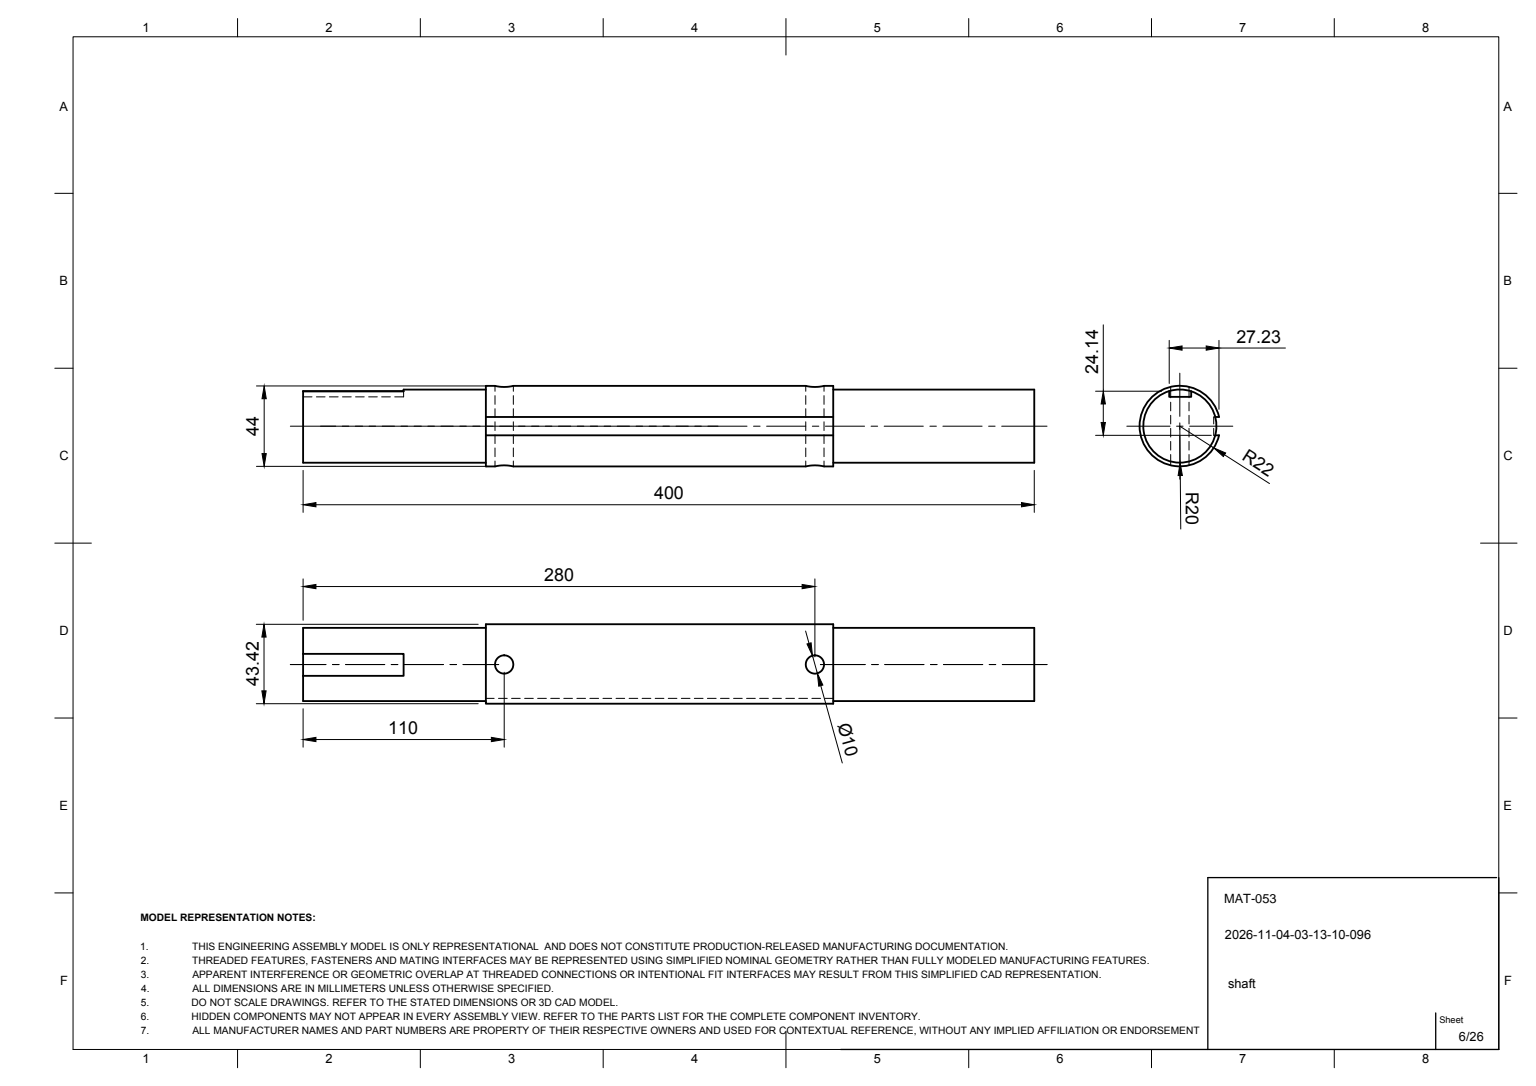
ISO-10303-21;
HEADER;
FILE_DESCRIPTION (('STEP AP214'),
    '1' );
FILE_NAME ('shaft.step',
    '2026-10-10T03:43:58',
    ( '' ),
    ( '' ),
    'SwSTEP 2.0',
    'SolidWorks 2026',
    '' );
FILE_SCHEMA (( 'AUTOMOTIVE_DESIGN' ));
ENDSEC;

DATA;
#13=ORIENTED_EDGE ( 'NONE', *, *, #19324, .T. ) ;
#42=CARTESIAN_POINT ( 'NONE',  ( 110.0000000000000284, 21.42428528562853174, 5.000000000000004441 ) ) ;
#241=DIRECTION ( 'NONE',  ( -0.000000000000000000, 1.000000000000000000, -0.000000000000000000 ) ) ;
#426=CARTESIAN_POINT ( 'NONE',  ( 283.3080539574502268, 21.67699184046404781, 3.763267418054555780 ) ) ;
#433=CARTESIAN_POINT ( 'NONE',  ( 105.1691917892558905, 21.96211590856092144, 1.300061720562576406 ) ) ;
#525=DIRECTION ( 'NONE',  ( -1.000000000000000000, -0.000000000000000000, -0.000000000000000000 ) ) ;
#698=ORIENTED_EDGE ( 'NONE', *, *, #41061, .T. ) ;
#760=FACE_OUTER_BOUND ( 'NONE', #64496, .T. ) ;
#778=PRODUCT_DEFINITION_CONTEXT ( 'detailed design', #31878, 'design' ) ;
#806=DIRECTION ( 'NONE',  ( 1.000000000000000000, 0.000000000000000000, 0.000000000000000000 ) ) ;
#952=CARTESIAN_POINT ( 'NONE',  ( 55.00000000000000000, 16.00000000000000000, 6.196318915105386793 ) ) ;
#960=EDGE_CURVE ( 'NONE', #18523, #30339, #59867, .T. ) ;
#977=B_SPLINE_CURVE_WITH_KNOTS ( 'NONE', 3,
 ( #65120, #65472, #59821, #42946, #10949, #11636, #44346, #64768, #17263, #27827, #54546, #27122, #33110, #17624, #39095, #33807, #59476, #6373, #37680, #53844, #16573, #60179, #26791, #12000, #33474, #60536, #54896, #6720, #5336, #11287, #48217, #28164, #59126, #42 ),
 .UNSPECIFIED., .F., .F.,
 ( 4, 2, 2, 2, 2, 2, 2, 2, 2, 2, 2, 2, 2, 2, 2, 2, 4 ),
 ( 0.01568356594869778006, 0.01666352729433787788, 0.01764348863997797917, 0.01862344998561807699, 0.01960341133125817828, 0.02058337267689827610, 0.02156333402253837739, 0.02254329536817847521, 0.02352325671381857303, 0.02450321805945867432, 0.02548317940509877561, 0.02646314075073887342, 0.02744310209637897124, 0.02842306344201907253, 0.02940302478765917035, 0.03038298613329926817, 0.03136294747893936946 ),
 .UNSPECIFIED. ) ;
#1162=EDGE_CURVE ( 'NONE', #19726, #7734, #16319, .T. ) ;
#1256=ORIENTED_EDGE ( 'NONE', *, *, #41395, .F. ) ;
#1285=EDGE_LOOP ( 'NONE', ( #47174, #10231, #18565, #33399, #41316, #43548, #36520, #6805, #23132 ) ) ;
#1304=CARTESIAN_POINT ( 'NONE',  ( 284.9999364138627129, -21.99998554860538391, -0.3278620034596229083 ) ) ;
#1329=EDGE_LOOP ( 'NONE', ( #45469, #25042, #63712, #61696 ) ) ;
#1555=VERTEX_POINT ( 'NONE', #50942 ) ;
#1629=ORIENTED_EDGE ( 'NONE', *, *, #37145, .F. ) ;
#1638=CARTESIAN_POINT ( 'NONE',  ( 108.3842135503130777, -21.48302731199173721, -4.742990268296093603 ) ) ;
#1878=( NAMED_UNIT ( * ) PLANE_ANGLE_UNIT ( ) SI_UNIT ( $, .RADIAN. ) );
#1903=ORIENTED_EDGE ( 'NONE', *, *, #43501, .F. ) ;
#1937=ORIENTED_EDGE ( 'NONE', *, *, #57039, .T. ) ;
#1939=CARTESIAN_POINT ( 'NONE',  ( 276.6934359423128740, 21.67676124233544499, 3.764605836381906379 ) ) ;
#1946=CARTESIAN_POINT ( 'NONE',  ( 110.0000000000000284, -21.42428528562853174, -5.000000000000004441 ) ) ;
#2003=CARTESIAN_POINT ( 'NONE',  ( 107.4937869665630359, -21.56868463414005177, -4.338918127843130357 ) ) ;
#2004=DIRECTION ( 'NONE',  ( 0.000000000000000000, 0.000000000000000000, 1.000000000000000000 ) ) ;
#2005=EDGE_CURVE ( 'NONE', #64974, #46266, #58883, .T. ) ;
#2193=DIRECTION ( 'NONE',  ( -0.000000000000000000, -0.000000000000000000, 1.000000000000000000 ) ) ;
#2217=PRESENTATION_STYLE_ASSIGNMENT (( #34229 ) ) ;
#2280=CARTESIAN_POINT ( 'NONE',  ( 278.3860478234813058, 21.48288568141374455, -4.743631494308814034 ) ) ;
#2460=EDGE_CURVE ( 'NONE', #11779, #61489, #23625, .T. ) ;
#2486=EDGE_CURVE ( 'NONE', #45063, #30339, #20404, .T. ) ;
#2511=DIRECTION ( 'NONE',  ( 1.000000000000000000, 0.000000000000000000, -0.000000000000000000 ) ) ;
#2544=EDGE_CURVE ( 'NONE', #45063, #35721, #38639, .T. ) ;
#2553=ORIENTED_EDGE ( 'NONE', *, *, #4045, .F. ) ;
#2560=FILL_AREA_STYLE_COLOUR ( '', #18851 ) ;
#2608=CARTESIAN_POINT ( 'NONE',  ( 275.6615829231344037, -21.85840048673442126, -2.507220999339073053 ) ) ;
#2648=FACE_BOUND ( 'NONE', #8178, .T. ) ;
#2649=FACE_OUTER_BOUND ( 'NONE', #33605, .T. ) ;
#2695=CARTESIAN_POINT ( 'NONE',  ( 283.9728608271481107, -21.78879854653021297, -3.053399776244554609 ) ) ;
#2795=LINE ( 'NONE', #34812, #43672 ) ;
#2969=CARTESIAN_POINT ( 'NONE',  ( 279.3426986656771760, 21.43197803755064967, 4.967354168418942173 ) ) ;
#3036=CARTESIAN_POINT ( 'NONE',  ( 108.7032261419851977, -21.46110313769845135, -4.839973237437577680 ) ) ;
#3041=ADVANCED_FACE ( 'NONE', ( #27935 ), #22661, .F. ) ;
#3300=CARTESIAN_POINT ( 'NONE',  ( 277.7808008216760527, -21.53681828009572996, -4.492424461587424034 ) ) ;
#3376=CARTESIAN_POINT ( 'NONE',  ( 109.6727132707902683, -21.42428528562852463, 5.000000000000001776 ) ) ;
#3443=DIRECTION ( 'NONE',  ( 0.000000000000000000, 0.000000000000000000, 1.000000000000000000 ) ) ;
#3562=VERTEX_POINT ( 'NONE', #44952 ) ;
#3581=VECTOR ( 'NONE', #57124, 1000.000000000000000 ) ;
#3756=DIRECTION ( 'NONE',  ( -1.000000000000000000, -0.000000000000000000, -0.000000000000000000 ) ) ;
#3846=AXIS2_PLACEMENT_3D ( 'NONE', #29576, #2511, #51044 ) ;
#3866=DIRECTION ( 'NONE',  ( -1.000000000000000000, -0.000000000000000000, -0.000000000000000000 ) ) ;
#3884=CARTESIAN_POINT ( 'NONE',  ( 280.0000000000000000, -21.42428528562853529, -4.999999999999990230 ) ) ;
#3905=EDGE_CURVE ( 'NONE', #17632, #45870, #3997, .T. ) ;
#3915=CARTESIAN_POINT ( 'NONE',  ( 110.3272854519634052, -21.42428528562852463, 5.000000000000005329 ) ) ;
#3997=LINE ( 'NONE', #8590, #30718 ) ;
#4045=EDGE_CURVE ( 'NONE', #19247, #46266, #9872, .T. ) ;
#4070=CYLINDRICAL_SURFACE ( 'NONE', #24334, 5.000000000000004441 ) ;
#4140=PRODUCT_DEFINITION_FORMATION_WITH_SPECIFIED_SOURCE ( 'ANY', '', #11948, .NOT_KNOWN. ) ;
#4184=FACE_OUTER_BOUND ( 'NONE', #48901, .T. ) ;
#4334=PLANE ( 'NONE',  #50993 ) ;
#4391=LINE ( 'NONE', #57852, #25285 ) ;
#4414=SHAPE_REPRESENTATION_RELATIONSHIP ( 'NONE' , 'NONE' ,  #63080, #69249 ) ;
#4473=AXIS2_PLACEMENT_3D ( 'NONE', #6447, #59199, #11358 ) ;
#4598=CARTESIAN_POINT ( 'NONE',  ( 111.2988829979105105, -21.46124357533057747, -4.839350883597181685 ) ) ;
#4658=ORIENTED_EDGE ( 'NONE', *, *, #37299, .T. ) ;
#4664=CARTESIAN_POINT ( 'NONE',  ( 283.7669346082183779, 21.75174821959686255, 3.303877464828343768 ) ) ;
#4882=ORIENTED_EDGE ( 'NONE', *, *, #49397, .T. ) ;
#5012=CARTESIAN_POINT ( 'NONE',  ( 281.6210066600216919, 21.48343462569976836, 4.741142292097720201 ) ) ;
#5108=SHAPE_DEFINITION_REPRESENTATION ( #35610, #63080 ) ;
#5161=CARTESIAN_POINT ( 'NONE',  ( -2.282530889443167084E-17, 4.999999999999999112, 21.42428528562853529 ) ) ;
#5181=DIRECTION ( 'NONE',  ( 0.000000000000000000, 0.000000000000000000, 1.000000000000000000 ) ) ;
#5320=EDGE_CURVE ( 'NONE', #30745, #45870, #39804, .T. ) ;
#5336=CARTESIAN_POINT ( 'NONE',  ( 112.2224082406587229, 21.53716320950900709, 4.490767689115658712 ) ) ;
#5532=CARTESIAN_POINT ( 'NONE',  ( 283.3053295232375035, -21.67655155662104249, 3.765949955696215046 ) ) ;
#5703=CARTESIAN_POINT ( 'NONE',  ( 108.3860478234812064, 21.48288568141374810, -4.743631494308838015 ) ) ;
#5723=ORIENTED_EDGE ( 'NONE', *, *, #10930, .F. ) ;
#5735=DIRECTION ( 'NONE',  ( 0.000000000000000000, 0.000000000000000000, 1.000000000000000000 ) ) ;
#5781=CARTESIAN_POINT ( 'NONE',  ( 278.7032261419851693, -21.46110313769844424, -4.839973237437567910 ) ) ;
#5862=DIRECTION ( 'NONE',  ( 1.000000000000000000, 0.000000000000000000, 0.000000000000000000 ) ) ;
#6165=VECTOR ( 'NONE', #60540, 1000.000000000000000 ) ;
#6220=CARTESIAN_POINT ( 'NONE',  ( 283.9749324730389048, -21.78918450429459241, 3.050527833458462457 ) ) ;
#6373=CARTESIAN_POINT ( 'NONE',  ( 115.0001299725262811, 22.00002953920830606, 0.3279435515783862276 ) ) ;
#6425=DIRECTION ( 'NONE',  ( 1.000000000000000000, -4.565061778886334783E-18, 0.000000000000000000 ) ) ;
#6447=CARTESIAN_POINT ( 'NONE',  ( 280.0000000000000000, -22.00000000000000000, 0.000000000000000000 ) ) ;
#6533=CARTESIAN_POINT ( 'NONE',  ( 100.0000000000000284, 5.000000000000000000, 18.50000000000000000 ) ) ;
#6624=ORIENTED_EDGE ( 'NONE', *, *, #2486, .F. ) ;
#6638=ORIENTED_EDGE ( 'NONE', *, *, #37538, .F. ) ;
#6667=DIRECTION ( 'NONE',  ( -0.000000000000000000, -0.000000000000000000, 1.000000000000000000 ) ) ;
#6688=VERTEX_POINT ( 'NONE', #35749 ) ;
#6720=CARTESIAN_POINT ( 'NONE',  ( 112.5093869099859063, 21.56904524376771093, 4.337160898883480442 ) ) ;
#6805=ORIENTED_EDGE ( 'NONE', *, *, #19457, .F. ) ;
#6911=ADVANCED_FACE ( 'NONE', ( #2649 ), #7925, .F. ) ;
#6981=CARTESIAN_POINT ( 'NONE',  ( -1.224646799147352468E-15, 19.01593100277520421, 6.196318915105386793 ) ) ;
#7100=DIRECTION ( 'NONE',  ( 0.000000000000000000, 0.000000000000000000, 1.000000000000000000 ) ) ;
#7112=LINE ( 'NONE', #56337, #35024 ) ;
#7189=LINE ( 'NONE', #7550, #25133 ) ;
#7272=CARTESIAN_POINT ( 'NONE',  ( 109.3447482101068289, -21.43190799616912301, -4.967656235065421200 ) ) ;
#7409=VECTOR ( 'NONE', #10719, 1000.000000000000000 ) ;
#7451=CARTESIAN_POINT ( 'NONE',  ( 290.0000000000000568, -5.000000000000000888, 18.50000000000000000 ) ) ;
#7549=CARTESIAN_POINT ( 'NONE',  ( 276.2352375355092704, -21.75137027410912438, -3.306356075928093219 ) ) ;
#7550=CARTESIAN_POINT ( 'NONE',  ( 100.0000000000000284, 5.000000000000000000, 18.50000000000000000 ) ) ;
#7561=CARTESIAN_POINT ( 'NONE',  ( 276.0273295991593727, 21.78875652052167311, 3.053836096979974268 ) ) ;
#7589=CYLINDRICAL_SURFACE ( 'NONE', #29305, 21.99999999999998579 ) ;
#7620=ORIENTED_EDGE ( 'NONE', *, *, #4045, .T. ) ;
#7627=CARTESIAN_POINT ( 'NONE',  ( 106.2352375355091993, -21.75137027410914214, -3.306356075928058580 ) ) ;
#7638=CARTESIAN_POINT ( 'NONE',  ( 280.6590877922806158, -21.43203852822545130, -4.967093445758824721 ) ) ;
#7649=ORIENTED_EDGE ( 'NONE', *, *, #12554, .T. ) ;
#7734=VERTEX_POINT ( 'NONE', #53587 ) ;
#7785=CARTESIAN_POINT ( 'NONE',  ( 290.0000000000000568, 5.000000000000000888, 19.36491673103706290 ) ) ;
#7811=EDGE_LOOP ( 'NONE', ( #57220, #47137, #53766, #56814, #30774 ) ) ;
#7870=CARTESIAN_POINT ( 'NONE',  ( 100.0000000000000284, 5.000000000000000000, 18.50000000000000000 ) ) ;
#7890=CARTESIAN_POINT ( 'NONE',  ( 276.0266963907629361, -21.78888161821124569, 3.052770673153777814 ) ) ;
#7898=CARTESIAN_POINT ( 'NONE',  ( 279.6730658560643974, 21.42428528562853884, -4.999999999999992006 ) ) ;
#7925=PLANE ( 'NONE',  #15187 ) ;
#7971=CARTESIAN_POINT ( 'NONE',  ( 284.9681307937125894, -21.99268844340181417, -0.6535439379101346535 ) ) ;
#8012=CIRCLE ( 'NONE', #30506, 20.00000000000000000 ) ;
#8178=EDGE_LOOP ( 'NONE', ( #4658, #42551 ) ) ;
#8298=CARTESIAN_POINT ( 'NONE',  ( 100.0000000000000284, -5.000000000000000000, 19.36491673103708777 ) ) ;
#8319=DIRECTION ( 'NONE',  ( 1.000000000000000000, 0.000000000000000000, 0.000000000000000000 ) ) ;
#8352=CARTESIAN_POINT ( 'NONE',  ( 0.000000000000000000, 0.000000000000000000, 20.00000000000000355 ) ) ;
#8462=VECTOR ( 'NONE', #33828, 1000.000000000000000 ) ;
#8471=ORIENTED_EDGE ( 'NONE', *, *, #21836, .T. ) ;
#8580=PLANE ( 'NONE',  #31900 ) ;
#8584=CARTESIAN_POINT ( 'NONE',  ( 284.3363611114016862, 21.85800776086857056, -2.510326265702884641 ) ) ;
#8587=CARTESIAN_POINT ( 'NONE',  ( 276.6944765335653074, -21.67660392622677534, -3.765493530430662261 ) ) ;
#8590=CARTESIAN_POINT ( 'NONE',  ( 0.000000000000000000, 19.01593100277521131, 6.196318915105386793 ) ) ;
#8661=CARTESIAN_POINT ( 'NONE',  ( 106.0266963907629645, -21.78888161821124925, 3.052770673153796466 ) ) ;
#8739=VERTEX_POINT ( 'NONE', #37345 ) ;
#8780=VECTOR ( 'NONE', #57937, 1000.000000000000000 ) ;
#8793=LINE ( 'NONE', #40782, #12943 ) ;
#8925=CARTESIAN_POINT ( 'NONE',  ( 284.8388692023054887, 21.96385131419673442, -1.300671796277831582 ) ) ;
#8929=CARTESIAN_POINT ( 'NONE',  ( 276.9483136162804726, -21.63883973695289242, 3.974316929722018443 ) ) ;
#8932=CARTESIAN_POINT ( 'NONE',  ( 107.7789859651022226, 21.53699436807883671, 4.491592093615980552 ) ) ;
#9239=ORIENTED_EDGE ( 'NONE', *, *, #46997, .F. ) ;
#9364=VECTOR ( 'NONE', #50767, 1000.000000000000000 ) ;
#9451=ORIENTED_EDGE ( 'NONE', *, *, #44658, .F. ) ;
#9675=CARTESIAN_POINT ( 'NONE',  ( -1.224646799147352468E-15, 16.00000000000000000, -5.803681084894614095 ) ) ;
#9698=( LENGTH_UNIT ( ) NAMED_UNIT ( * ) SI_UNIT ( .MILLI., .METRE. ) );
#9872=B_SPLINE_CURVE_WITH_KNOTS ( 'NONE', 3,
 ( #24424, #19830, #68366, #36349, #19126, #8932, #30379, #57801, #45866, #62035, #41283, #62742, #35312, #14546, #57457, #433, #42654, #64111, #53189, #64455, #53541, #59509, #58475, #10633, #64808, #48945, #53880, #42314, #37365, #36701, #16608, #5703, #21207, #9965, #31418, #27160 ),
 .UNSPECIFIED., .F., .F.,
 ( 4, 2, 2, 2, 2, 2, 2, 2, 2, 2, 2, 2, 2, 2, 2, 2, 2, 4 ),
 ( 0.000000000000000000, 0.0009802228717936162412, 0.001960445743587232482, 0.002940668615380848724, 0.003920891487174464965, 0.004901114358968081640, 0.005881337230761697447, 0.006371448666658505351, 0.006861560102555313255, 0.007841782974348921256, 0.008822005846142528390, 0.009802228717936137259, 0.01078245158972974439, 0.01176267446152335153, 0.01274289733331695866, 0.01372312020511056579, 0.01470334307690417466, 0.01568356594869778006 ),
 .UNSPECIFIED. ) ;
#9920=CARTESIAN_POINT ( 'NONE',  ( 100.0000000000000284, 5.000000000000000000, 18.50000000000000000 ) ) ;
#9959=CARTESIAN_POINT ( 'NONE',  ( 284.8405205227987835, 21.96421596965998901, 1.294720749503649015 ) ) ;
#9965=CARTESIAN_POINT ( 'NONE',  ( 109.3411025683418529, 21.43200632497275038, -4.967238636669211616 ) ) ;
#9990=CARTESIAN_POINT ( 'NONE',  ( 55.00000000000000000, 16.00000000000000000, -5.803681084894614095 ) ) ;
#10222=DIRECTION ( 'NONE',  ( 1.000000000000000000, 0.000000000000000000, 0.000000000000000000 ) ) ;
#10231=ORIENTED_EDGE ( 'NONE', *, *, #2486, .T. ) ;
#10333=EDGE_CURVE ( 'NONE', #3562, #45063, #42398, .T. ) ;
#10344=DIRECTION ( 'NONE',  ( -1.000000000000000000, -0.000000000000000000, -0.000000000000000000 ) ) ;
#10458=CARTESIAN_POINT ( 'NONE',  ( 280.3272854519634052, -21.42428528562853529, 4.999999999999992895 ) ) ;
#10575=CARTESIAN_POINT ( 'NONE',  ( 100.0000000000000284, -5.000000000000000000, 18.50000000000000000 ) ) ;
#10627=CARTESIAN_POINT ( 'NONE',  ( 284.4933711091047712, 21.89007574053286120, 2.217281872662929754 ) ) ;
#10633=CARTESIAN_POINT ( 'NONE',  ( 105.5073993722360655, 21.88991381840459383, -2.219103374846306931 ) ) ;
#10637=ORIENTED_EDGE ( 'NONE', *, *, #64391, .T. ) ;
#10719=DIRECTION ( 'NONE',  ( -1.000000000000000000, -0.000000000000000000, -0.000000000000000000 ) ) ;
#10724=DIRECTION ( 'NONE',  ( 0.000000000000000000, 0.000000000000000000, 1.000000000000000000 ) ) ;
#10811=CARTESIAN_POINT ( 'NONE',  ( 281.6139602183311013, -21.48286796535249721, 4.743729604094155228 ) ) ;
#10833=DIRECTION ( 'NONE',  ( -1.000000000000000000, -0.000000000000000000, -0.000000000000000000 ) ) ;
#10930=EDGE_CURVE ( 'NONE', #11717, #61489, #53330, .T. ) ;
#10949=CARTESIAN_POINT ( 'NONE',  ( 111.6145892210130199, 21.48294702482179375, -4.743341903180122721 ) ) ;
#11120=EDGE_CURVE ( 'NONE', #16987, #44224, #64599, .T. ) ;
#11287=CARTESIAN_POINT ( 'NONE',  ( 111.6210066600218198, 21.48343462569976836, 4.741142292097735300 ) ) ;
#11318=CARTESIAN_POINT ( 'NONE',  ( 282.5093869099858921, 21.56904524376771093, 4.337160898883471560 ) ) ;
#11358=DIRECTION ( 'NONE',  ( 0.000000000000000000, 0.000000000000000000, 1.000000000000000000 ) ) ;
#11550=EDGE_LOOP ( 'NONE', ( #12840, #44077, #49586, #1937 ) ) ;
#11636=CARTESIAN_POINT ( 'NONE',  ( 112.2165994398967399, 21.53656025449836164, -4.493648593974088890 ) ) ;
#11717=VERTEX_POINT ( 'NONE', #54907 ) ;
#11775=ORIENTED_EDGE ( 'NONE', *, *, #59603, .T. ) ;
#11779=VERTEX_POINT ( 'NONE', #7785 ) ;
#11887=DIRECTION ( 'NONE',  ( 0.000000000000000000, 0.000000000000000000, 1.000000000000000000 ) ) ;
#11931=ORIENTED_EDGE ( 'NONE', *, *, #43815, .F. ) ;
#11948=PRODUCT ( 'shaft', 'shaft', '', ( #64547 ) ) ;
#12000=CARTESIAN_POINT ( 'NONE',  ( 113.9761838721218368, 21.78940454476515853, 3.049139182071525678 ) ) ;
#12295=AXIS2_PLACEMENT_3D ( 'NONE', #53675, #32581, #15711 ) ;
#12312=CYLINDRICAL_SURFACE ( 'NONE', #63138, 19.99999999999998934 ) ;
#12401=CARTESIAN_POINT ( 'NONE',  ( 100.0000000000000284, -5.000000000000000000, 18.50000000000000000 ) ) ;
#12409=EDGE_LOOP ( 'NONE', ( #44300, #52366 ) ) ;
#12521=EDGE_LOOP ( 'NONE', ( #53310, #62518, #64465, #27014 ) ) ;
#12544=CARTESIAN_POINT ( 'NONE',  ( 400.0000000000000000, 2.449293598294706513E-15, -20.00000000000000000 ) ) ;
#12554=EDGE_CURVE ( 'NONE', #59695, #25409, #43625, .T. ) ;
#12563=CARTESIAN_POINT ( 'NONE',  ( 290.0000000000000568, 5.000000000000000888, 18.50000000000000000 ) ) ;
#12659=ORIENTED_EDGE ( 'NONE', *, *, #55904, .T. ) ;
#12661=FACE_OUTER_BOUND ( 'NONE', #14836, .T. ) ;
#12799=AXIS2_PLACEMENT_3D ( 'NONE', #37614, #63674, #58717 ) ;
#12834=CARTESIAN_POINT ( 'NONE',  ( 278.6977768404063340, 21.46141967451381305, -4.838576272177869342 ) ) ;
#12835=CARTESIAN_POINT ( 'NONE',  ( 290.0000000000000568, 5.000000000000000888, 18.50000000000000000 ) ) ;
#12840=ORIENTED_EDGE ( 'NONE', *, *, #53641, .F. ) ;
#12879=AXIS2_PLACEMENT_3D ( 'NONE', #16393, #38187, #37846 ) ;
#12922=LINE ( 'NONE', #12563, #63487 ) ;
#12943=VECTOR ( 'NONE', #47430, 1000.000000000000000 ) ;
#12992=ORIENTED_EDGE ( 'NONE', *, *, #26604, .F. ) ;
#13121=SURFACE_STYLE_FILL_AREA ( #50050 ) ;
#13157=VERTEX_POINT ( 'NONE', #62870 ) ;
#13180=CARTESIAN_POINT ( 'NONE',  ( 275.1691917892559331, 21.96211590856092144, 1.300061720562569301 ) ) ;
#13299=ADVANCED_FACE ( 'NONE', ( #32241 ), #37502, .F. ) ;
#13361=CARTESIAN_POINT ( 'NONE',  ( 0.000000000000000000, 0.000000000000000000, 0.000000000000000000 ) ) ;
#13509=CARTESIAN_POINT ( 'NONE',  ( 283.0520942216416529, 21.63891660051134380, -3.973857610334881496 ) ) ;
#13513=CARTESIAN_POINT ( 'NONE',  ( 276.2372751229154346, -21.75101418369302309, 3.308700176549365324 ) ) ;
#13522=EDGE_CURVE ( 'NONE', #46266, #19247, #977, .T. ) ;
#13549=FACE_OUTER_BOUND ( 'NONE', #11550, .T. ) ;
#13848=CARTESIAN_POINT ( 'NONE',  ( 278.3885044869534227, -21.48423713950020897, 4.736025848076669931 ) ) ;
#13849=DIRECTION ( 'NONE',  ( -0.000000000000000000, -0.000000000000000000, 1.000000000000000000 ) ) ;
#13930=( NAMED_UNIT ( * ) PLANE_ANGLE_UNIT ( ) SI_UNIT ( $, .RADIAN. ) );
#13991=ORIENTED_EDGE ( 'NONE', *, *, #25374, .F. ) ;
#13997=CARTESIAN_POINT ( 'NONE',  ( 100.0000000000000284, 0.000000000000000000, 0.000000000000000000 ) ) ;
#14199=CARTESIAN_POINT ( 'NONE',  ( 281.6145892210130341, 21.48294702482179730, -4.743341903180106733 ) ) ;
#14202=CARTESIAN_POINT ( 'NONE',  ( 275.1608565259479633, -21.96391085485757699, -1.300312621757654608 ) ) ;
#14244=DIRECTION ( 'NONE',  ( -1.000000000000000000, -0.000000000000000000, -0.000000000000000000 ) ) ;
#14278=CARTESIAN_POINT ( 'NONE',  ( 108.7020975237396812, -21.46299323290192618, 4.831387770023936490 ) ) ;
#14334=ORIENTED_EDGE ( 'NONE', *, *, #2460, .F. ) ;
#14427=B_SPLINE_CURVE_WITH_KNOTS ( 'NONE', 3,
 ( #28647, #17751, #39206, #5781, #49027, #3300, #40244, #29337, #8587, #7549, #56411, #2608, #24067, #50451, #14202, #30036, #57116, #29008, #50789, #39892, #61688, #56073, #29682, #7890, #13513, #51499, #8929, #34968, #61349, #45511, #13848, #24761, #66995, #46194, #23718, #61000 ),
 .UNSPECIFIED., .F., .F.,
 ( 4, 2, 2, 2, 2, 2, 2, 2, 2, 2, 2, 2, 2, 2, 2, 2, 2, 4 ),
 ( 0.02352539391595311752, 0.02450549414544721943, 0.02548559437494132135, 0.02646569460443541980, 0.02744579483392952171, 0.02842589506342362016, 0.02940599529291772207, 0.03038609552241182052, 0.03136619575190591896, 0.03234629598140002088, 0.03332639621089411586, 0.03430649644038821777, 0.03528659666988231969, 0.03626669689937642160, 0.03724679712887052352, 0.03773684724361749815, 0.03822689735836447278, 0.03920699758785825551 ),
 .UNSPECIFIED. ) ;
#14472=CARTESIAN_POINT ( 'NONE',  ( 110.3299582524531957, -21.42428528562853174, -5.000000000000005329 ) ) ;
#14546=CARTESIAN_POINT ( 'NONE',  ( 105.3198800741404284, 21.92942769035742501, 1.767193244627911719 ) ) ;
#14615=CARTESIAN_POINT ( 'NONE',  ( 108.2349883415519258, -21.49634503089637150, 4.680941717099545762 ) ) ;
#14836=EDGE_LOOP ( 'NONE', ( #57828, #66420, #40388, #21025, #22944 ) ) ;
#15084=CARTESIAN_POINT ( 'NONE',  ( -1.224646799147352468E-15, 0.000000000000000000, 0.000000000000000000 ) ) ;
#15160=CARTESIAN_POINT ( 'NONE',  ( 114.9999364138626703, -21.99998554860538391, -0.3278620034596400612 ) ) ;
#15187=AXIS2_PLACEMENT_3D ( 'NONE', #6533, #50832, #24112 ) ;
#15362=DIRECTION ( 'NONE',  ( -0.000000000000000000, -0.000000000000000000, -1.000000000000000000 ) ) ;
#15541=DIRECTION ( 'NONE',  ( -0.000000000000000000, -0.000000000000000000, 1.000000000000000000 ) ) ;
#15563=CARTESIAN_POINT ( 'NONE',  ( 110.0000000000000284, 21.42428528562853529, -5.000000000000004441 ) ) ;
#15569=ORIENTED_EDGE ( 'NONE', *, *, #5320, .T. ) ;
#15582=CARTESIAN_POINT ( 'NONE',  ( 281.3030933484816956, 21.46146164524276045, 4.838392277045652001 ) ) ;
#15652=DIRECTION ( 'NONE',  ( 0.000000000000000000, 0.000000000000000000, 1.000000000000000000 ) ) ;
#15711=DIRECTION ( 'NONE',  ( 0.000000000000000000, 0.000000000000000000, -1.000000000000000000 ) ) ;
#15866=PLANE ( 'NONE',  #44385 ) ;
#16085=CARTESIAN_POINT ( 'NONE',  ( 280.0000000000000000, -21.42428528562853884, 4.999999999999990230 ) ) ;
#16188=DIRECTION ( 'NONE',  ( -0.000000000000000000, 1.000000000000000000, -0.000000000000000000 ) ) ;
#16302=FACE_OUTER_BOUND ( 'NONE', #31686, .T. ) ;
#16319=LINE ( 'NONE', #9675, #20560 ) ;
#16323=AXIS2_PLACEMENT_3D ( 'NONE', #34529, #19022, #67563 ) ;
#16393=CARTESIAN_POINT ( 'NONE',  ( 0.000000000000000000, 16.00000000000000000, 0.000000000000000000 ) ) ;
#16573=CARTESIAN_POINT ( 'NONE',  ( 114.7436796776308086, 21.94282408638629889, 1.613761426918485897 ) ) ;
#16608=CARTESIAN_POINT ( 'NONE',  ( 107.7821011353898939, 21.53668059256674283, -4.493084242282758822 ) ) ;
#16775=CARTESIAN_POINT ( 'NONE',  ( 283.0516338319616807, -21.63887047452759305, 3.974065166673101057 ) ) ;
#16938=VECTOR ( 'NONE', #27193, 1000.000000000000000 ) ;
#16983=ADVANCED_FACE ( 'NONE', ( #29841 ), #39356, .F. ) ;
#16987=VERTEX_POINT ( 'NONE', #17548 ) ;
#17263=CARTESIAN_POINT ( 'NONE',  ( 113.3030319151915251, 21.67621409537482080, -3.767785295203596618 ) ) ;
#17377=DIRECTION ( 'NONE',  ( 1.000000000000000000, 0.000000000000000000, 0.000000000000000000 ) ) ;
#17548=CARTESIAN_POINT ( 'NONE',  ( 280.0000000000000000, -21.42428528562853884, 4.999999999999990230 ) ) ;
#17624=CARTESIAN_POINT ( 'NONE',  ( 114.7429971699385192, 21.94267019860760470, -1.616224894600706952 ) ) ;
#17632=VERTEX_POINT ( 'NONE', #57026 ) ;
#17682=AXIS2_PLACEMENT_3D ( 'NONE', #44552, #28726, #2004 ) ;
#17748=MECHANICAL_DESIGN_GEOMETRIC_PRESENTATION_REPRESENTATION('',(#58158),#57014);
#17751=CARTESIAN_POINT ( 'NONE',  ( 279.6700404598698242, -21.42428528562853529, -4.999999999999990230 ) ) ;
#17798=DIRECTION ( 'NONE',  ( 0.000000000000000000, 0.000000000000000000, 1.000000000000000000 ) ) ;
#17834=CARTESIAN_POINT ( 'NONE',  ( 284.8388622179743948, -21.96384902133207362, 1.301157935232950980 ) ) ;
#18382=( NAMED_UNIT ( * ) SI_UNIT ( $, .STERADIAN. ) SOLID_ANGLE_UNIT ( ) );
#18448=CARTESIAN_POINT ( 'NONE',  ( 278.7021502624938876, 21.46117544541993638, 4.839652729015472943 ) ) ;
#18507=EDGE_CURVE ( 'NONE', #7734, #18523, #23129, .T. ) ;
#18516=CARTESIAN_POINT ( 'NONE',  ( 106.0271074675581673, -21.78879721737672526, -3.053546265906987855 ) ) ;
#18523=VERTEX_POINT ( 'NONE', #18888 ) ;
#18565=ORIENTED_EDGE ( 'NONE', *, *, #960, .F. ) ;
#18693=CARTESIAN_POINT ( 'NONE',  ( 0.000000000000000000, 0.000000000000000000, 19.99999999999998934 ) ) ;
#18703=CYLINDRICAL_SURFACE ( 'NONE', #21096, 4.999999999999990230 ) ;
#18746=CARTESIAN_POINT ( 'NONE',  ( 290.0000000000000568, 0.000000000000000000, 0.000000000000000000 ) ) ;
#18792=CARTESIAN_POINT ( 'NONE',  ( 276.9495076362458121, 21.63869423720476703, 3.975053342410747259 ) ) ;
#18851=COLOUR_RGB ( '',0.7921568627450980005, 0.8196078431372548767, 0.9333333333333333481 ) ;
#18888=CARTESIAN_POINT ( 'NONE',  ( -1.224646799147352468E-15, 19.13941707223175825, -5.803681084894614095 ) ) ;
#19022=DIRECTION ( 'NONE',  ( 0.000000000000000000, 0.000000000000000000, 1.000000000000000000 ) ) ;
#19115=UNCERTAINTY_MEASURE_WITH_UNIT (LENGTH_MEASURE( 1.000000000000000082E-05 ), #9698, 'distance_accuracy_value', 'NONE');
#19118=ADVANCED_FACE ( 'NONE', ( #43691 ), #65169, .F. ) ;
#19126=CARTESIAN_POINT ( 'NONE',  ( 108.3839814017204617, 21.48303375171747120, 4.742972355882020707 ) ) ;
#19132=CARTESIAN_POINT ( 'NONE',  ( 100.0000000000000284, -5.000000000000000000, 21.42428528562851753 ) ) ;
#19170=CARTESIAN_POINT ( 'NONE',  ( -1.224646799147352468E-15, 0.000000000000000000, 0.000000000000000000 ) ) ;
#19247=VERTEX_POINT ( 'NONE', #21813 ) ;
#19271=EDGE_LOOP ( 'NONE', ( #7620, #21554 ) ) ;
#19304=VECTOR ( 'NONE', #3756, 1000.000000000000000 ) ;
#19324=EDGE_CURVE ( 'NONE', #54597, #6688, #24186, .T. ) ;
#19392=CARTESIAN_POINT ( 'NONE',  ( 113.9728608271480965, -21.78879854653021297, -3.053399776244579478 ) ) ;
#19457=EDGE_CURVE ( 'NONE', #60501, #30745, #47010, .T. ) ;
#19466=CARTESIAN_POINT ( 'NONE',  ( 281.3012118866374180, 21.46131765974229566, -4.839032743736807696 ) ) ;
#19724=CARTESIAN_POINT ( 'NONE',  ( 290.0000000000000568, 5.000000000000000888, 18.50000000000000000 ) ) ;
#19726=VERTEX_POINT ( 'NONE', #9990 ) ;
#19742=CARTESIAN_POINT ( 'NONE',  ( 114.3366190915103289, -21.85805078441902793, -2.510101233139118815 ) ) ;
#19830=CARTESIAN_POINT ( 'NONE',  ( 109.6684666882775474, 21.42428528562853529, 5.000000000000007105 ) ) ;
#19901=CARTESIAN_POINT ( 'NONE',  ( 104.9997958498911288, -22.00004639774357429, -0.3283548106454132198 ) ) ;
#19974=CARTESIAN_POINT ( 'NONE',  ( 100.0000000000000284, -5.000000000000000000, 18.50000000000000000 ) ) ;
#20069=B_SPLINE_CURVE_WITH_KNOTS ( 'NONE', 3,
 ( #60659, #35318, #2969, #18448, #29345, #33939, #24080, #18792, #1939, #61357, #7561, #45173, #29019, #44833, #50459, #13180, #51158, #30046, #40251, #51506, #67003, #24431, #61697, #23396, #46203, #39902, #66314, #28658, #34647, #34976, #56083, #2280, #12834, #56420, #7898, #50799 ),
 .UNSPECIFIED., .F., .F.,
 ( 4, 2, 2, 2, 2, 2, 2, 2, 2, 2, 2, 2, 2, 2, 2, 2, 2, 4 ),
 ( 0.000000000000000000, 0.0009802228717936478999, 0.001960445743587295800, 0.002940668615380943266, 0.003920891487174591600, 0.004901114358968239500, 0.005881337230761886532, 0.006371448666658678824, 0.006861560102555471982, 0.007841782974349056565, 0.008822005846142642882, 0.009802228717936227465, 0.01078245158972981205, 0.01176267446152339316, 0.01274289733331697774, 0.01372312020511056059, 0.01470334307690414517, 0.01568356594869772802 ),
 .UNSPECIFIED. ) ;
#20093=CARTESIAN_POINT ( 'NONE',  ( 114.9673805781175133, -21.99252023018708968, 0.6578219585121953816 ) ) ;
#20235=CARTESIAN_POINT ( 'NONE',  ( 109.3475734619033659, -21.43178884250801275, 4.968175626252066657 ) ) ;
#20355=EDGE_LOOP ( 'NONE', ( #57247, #41936, #42444, #59571 ) ) ;
#20375=CARTESIAN_POINT ( 'NONE',  ( 400.0000000000000000, 0.000000000000000000, 0.000000000000000000 ) ) ;
#20404=LINE ( 'NONE', #30978, #20666 ) ;
#20425=CARTESIAN_POINT ( 'NONE',  ( 113.0494652463580536, -21.63856170200817530, -3.975743201777092839 ) ) ;
#20432=DIRECTION ( 'NONE',  ( -0.000000000000000000, 0.000000000000000000, 1.000000000000000000 ) ) ;
#20495=ADVANCED_FACE ( 'NONE', ( #38270 ), #32317, .T. ) ;
#20560=VECTOR ( 'NONE', #10344, 1000.000000000000000 ) ;
#20572=CARTESIAN_POINT ( 'NONE',  ( 105.2579757425518210, -21.94246241598115432, 1.618793836905549233 ) ) ;
#20573=EDGE_CURVE ( 'NONE', #29607, #19726, #68810, .T. ) ;
#20666=VECTOR ( 'NONE', #32008, 1000.000000000000000 ) ;
#20758=CIRCLE ( 'NONE', #43183, 19.99999999999998934 ) ;
#20767=ORIENTED_EDGE ( 'NONE', *, *, #46997, .T. ) ;
#20775=CARTESIAN_POINT ( 'NONE',  ( 113.0516338319616665, -21.63887047452759305, 3.974065166673112603 ) ) ;
#21025=ORIENTED_EDGE ( 'NONE', *, *, #50272, .F. ) ;
#21096=AXIS2_PLACEMENT_3D ( 'NONE', #24338, #28917, #7100 ) ;
#21207=CARTESIAN_POINT ( 'NONE',  ( 108.6977768404062914, 21.46141967451380950, -4.838576272177880000 ) ) ;
#21463=LINE ( 'NONE', #42907, #54066 ) ;
#21554=ORIENTED_EDGE ( 'NONE', *, *, #13522, .T. ) ;
#21700=CARTESIAN_POINT ( 'NONE',  ( 110.0000000000000284, -22.00000000000000000, 0.000000000000000000 ) ) ;
#21813=CARTESIAN_POINT ( 'NONE',  ( 110.0000000000000284, 21.42428528562853174, 5.000000000000004441 ) ) ;
#21836=EDGE_CURVE ( 'NONE', #6688, #42114, #45842, .T. ) ;
#21951=CARTESIAN_POINT ( 'NONE',  ( 110.0000000000000284, -22.00000000000000000, -5.000000000000004441 ) ) ;
#22402=DIRECTION ( 'NONE',  ( 0.000000000000000000, 0.000000000000000000, 1.000000000000000000 ) ) ;
#22405=DIRECTION ( 'NONE',  ( -0.000000000000000000, 1.000000000000000000, -0.000000000000000000 ) ) ;
#22445=DIRECTION ( 'NONE',  ( -1.000000000000000000, -0.000000000000000000, -0.000000000000000000 ) ) ;
#22661=PLANE ( 'NONE',  #60989 ) ;
#22682=ADVANCED_FACE ( 'NONE', ( #56758 ), #8580, .F. ) ;
#22698=ADVANCED_FACE ( 'NONE', ( #46892 ), #4334, .F. ) ;
#22755=CARTESIAN_POINT ( 'NONE',  ( 284.8387163486434588, -21.96381563589838493, -1.302408292197359208 ) ) ;
#22906=ORIENTED_EDGE ( 'NONE', *, *, #30192, .F. ) ;
#22944=ORIENTED_EDGE ( 'NONE', *, *, #35331, .F. ) ;
#22951=DIRECTION ( 'NONE',  ( 1.000000000000000000, 0.000000000000000000, 0.000000000000000000 ) ) ;
#23102=CYLINDRICAL_SURFACE ( 'NONE', #17682, 20.00000000000000355 ) ;
#23129=LINE ( 'NONE', #62842, #27176 ) ;
#23132=ORIENTED_EDGE ( 'NONE', *, *, #50272, .T. ) ;
#23332=VECTOR ( 'NONE', #64750, 1000.000000000000000 ) ;
#23344=DIRECTION ( 'NONE',  ( 0.000000000000000000, 0.000000000000000000, -1.000000000000000000 ) ) ;
#23396=CARTESIAN_POINT ( 'NONE',  ( 275.5073993722361934, 21.88991381840460448, -2.219103374846307375 ) ) ;
#23459=CARTESIAN_POINT ( 'NONE',  ( 106.9490892766209527, -21.63874093657134878, -3.974828052515719801 ) ) ;
#23616=CARTESIAN_POINT ( 'NONE',  ( 110.0000000000000284, -21.42428528562853529, 5.000000000000004441 ) ) ;
#23625=LINE ( 'NONE', #19724, #37479 ) ;
#23653=ORIENTED_EDGE ( 'NONE', *, *, #2005, .T. ) ;
#23718=CARTESIAN_POINT ( 'NONE',  ( 279.6727132707902115, -21.42428528562853174, 4.999999999999985789 ) ) ;
#23727=CIRCLE ( 'NONE', #61922, 19.99999999999997868 ) ;
#23848=ORIENTED_EDGE ( 'NONE', *, *, #24705, .F. ) ;
#23941=AXIS2_PLACEMENT_3D ( 'NONE', #38199, #34339, #44529 ) ;
#24053=ORIENTED_EDGE ( 'NONE', *, *, #59603, .F. ) ;
#24067=CARTESIAN_POINT ( 'NONE',  ( 275.5080822241899909, -21.88977794987917491, -2.220096651196673765 ) ) ;
#24080=CARTESIAN_POINT ( 'NONE',  ( 277.4922189950061693, 21.56887920590509111, 4.337924292484275135 ) ) ;
#24112=DIRECTION ( 'NONE',  ( -1.000000000000000000, -4.565061778886334783E-18, 0.000000000000000000 ) ) ;
#24159=CARTESIAN_POINT ( 'NONE',  ( 282.2220340837702679, -21.53708152545855725, -4.491189304432787743 ) ) ;
#24186=LINE ( 'NONE', #35073, #50734 ) ;
#24247=DIRECTION ( 'NONE',  ( -0.000000000000000000, -0.000000000000000000, 1.000000000000000000 ) ) ;
#24265=DIRECTION ( 'NONE',  ( 0.000000000000000000, 0.000000000000000000, 1.000000000000000000 ) ) ;
#24289=B_SPLINE_CURVE_WITH_KNOTS ( 'NONE', 3,
 ( #45238, #50174, #7272, #3036, #1638, #28725, #2003, #23459, #34361, #7627, #18516, #56845, #42037, #31486, #36769, #41694, #19901, #68759, #67748, #46972, #20572, #36075, #30450, #8661, #63154, #57875, #41009, #30801, #46623, #14615, #68098, #14278, #69101, #20235, #3376, #68430 ),
 .UNSPECIFIED., .F., .F.,
 ( 4, 2, 2, 2, 2, 2, 2, 2, 2, 2, 2, 2, 2, 2, 2, 2, 2, 4 ),
 ( 0.02352539391595309323, 0.02450549414544716739, 0.02548559437494124155, 0.02646569460443531571, 0.02744579483392938987, 0.02842589506342346750, 0.02940599529291754166, 0.03038609552241161235, 0.03136619575190568998, 0.03234629598139976414, 0.03332639621089383830, 0.03430649644038791246, 0.03528659666988198662, 0.03626669689937606078, 0.03724679712887013494, 0.03773684724361715120, 0.03822689735836416747, 0.03920699758785820693 ),
 .UNSPECIFIED. ) ;
#24334=AXIS2_PLACEMENT_3D ( 'NONE', #25188, #25534, #15652 ) ;
#24338=CARTESIAN_POINT ( 'NONE',  ( 280.0000000000000000, -22.00000000000000000, 0.000000000000000000 ) ) ;
#24424=CARTESIAN_POINT ( 'NONE',  ( 110.0000000000000284, 21.42428528562853174, 5.000000000000004441 ) ) ;
#24431=CARTESIAN_POINT ( 'NONE',  ( 275.1608908971991809, 21.96390383200032304, -1.300086469598740635 ) ) ;
#24519=DIRECTION ( 'NONE',  ( -0.000000000000000000, 1.000000000000000000, -0.000000000000000000 ) ) ;
#24582=DIRECTION ( 'NONE',  ( 0.000000000000000000, 0.000000000000000000, -1.000000000000000000 ) ) ;
#24688=CARTESIAN_POINT ( 'NONE',  ( 111.3018128478065876, -21.46140473645479929, 4.838640910132746775 ) ) ;
#24705=EDGE_CURVE ( 'NONE', #59695, #54597, #12922, .T. ) ;
#24753=CARTESIAN_POINT ( 'NONE',  ( 55.00000000000000000, 16.00000000000000000, -5.803681084894614095 ) ) ;
#24761=CARTESIAN_POINT ( 'NONE',  ( 278.7020975237396669, -21.46299323290192262, 4.831387770023922279 ) ) ;
#24860=DIRECTION ( 'NONE',  ( -0.000000000000000000, 1.000000000000000000, -0.000000000000000000 ) ) ;
#24962=CLOSED_SHELL ( 'NONE', ( #33525, #28753, #47220, #56709, #44214, #38210, #22698, #50856, #13299, #20495, #38344, #69389, #48124, #22682, #16983, #65683, #42644, #3041, #6911, #19118, #38202, #27699 ) ) ;
#25034=CARTESIAN_POINT ( 'NONE',  ( 113.9749324730388622, -21.78918450429459241, 3.050527833458433591 ) ) ;
#25042=ORIENTED_EDGE ( 'NONE', *, *, #1162, .F. ) ;
#25133=VECTOR ( 'NONE', #13849, 1000.000000000000000 ) ;
#25188=CARTESIAN_POINT ( 'NONE',  ( 110.0000000000000284, -22.00000000000000000, 0.000000000000000000 ) ) ;
#25285=VECTOR ( 'NONE', #30430, 1000.000000000000000 ) ;
#25313=AXIS2_PLACEMENT_3D ( 'NONE', #51311, #24582, #65752 ) ;
#25319=ORIENTED_EDGE ( 'NONE', *, *, #35331, .T. ) ;
#25374=EDGE_CURVE ( 'NONE', #61489, #8739, #53412, .T. ) ;
#25409=VERTEX_POINT ( 'NONE', #42323 ) ;
#25534=DIRECTION ( 'NONE',  ( -0.000000000000000000, 1.000000000000000000, -0.000000000000000000 ) ) ;
#25577=EDGE_LOOP ( 'NONE', ( #4882, #38723 ) ) ;
#25610=ORIENTED_EDGE ( 'NONE', *, *, #11120, .F. ) ;
#25727=CARTESIAN_POINT ( 'NONE',  ( 114.3366674800923732, -21.85806848808613267, 2.509805449637990016 ) ) ;
#25798=CARTESIAN_POINT ( 'NONE',  ( 282.2165994398968110, 21.53656025449836520, -4.493648593974075567 ) ) ;
#25868=ORIENTED_EDGE ( 'NONE', *, *, #51003, .F. ) ;
#26064=CARTESIAN_POINT ( 'NONE',  ( 114.8388622179743805, -21.96384902133207362, 1.301157935232943430 ) ) ;
#26564=LINE ( 'NONE', #69113, #7409 ) ;
#26604=EDGE_CURVE ( 'NONE', #3562, #11717, #47522, .T. ) ;
#26770=CIRCLE ( 'NONE', #66119, 19.99999999999998934 ) ;
#26791=CARTESIAN_POINT ( 'NONE',  ( 114.3399910931246950, 21.85871988289598988, 2.504349266409138242 ) ) ;
#26813=DIRECTION ( 'NONE',  ( -0.000000000000000000, 0.000000000000000000, 1.000000000000000000 ) ) ;
#26857=CARTESIAN_POINT ( 'NONE',  ( 290.0000000000000568, 0.000000000000000000, 0.000000000000000000 ) ) ;
#27014=ORIENTED_EDGE ( 'NONE', *, *, #13522, .F. ) ;
#27105=DIRECTION ( 'NONE',  ( -1.000000000000000000, 0.000000000000000000, -0.000000000000000000 ) ) ;
#27122=CARTESIAN_POINT ( 'NONE',  ( 114.3363611114016578, 21.85800776086857411, -2.510326265702867765 ) ) ;
#27160=CARTESIAN_POINT ( 'NONE',  ( 110.0000000000000284, 21.42428528562853529, -5.000000000000004441 ) ) ;
#27176=VECTOR ( 'NONE', #24860, 1000.000000000000000 ) ;
#27193=DIRECTION ( 'NONE',  ( 0.000000000000000000, 0.000000000000000000, 1.000000000000000000 ) ) ;
#27281=ORIENTED_EDGE ( 'NONE', *, *, #51556, .F. ) ;
#27474=ORIENTED_EDGE ( 'NONE', *, *, #55904, .F. ) ;
#27500=CARTESIAN_POINT ( 'NONE',  ( 55.00000000000000000, 16.00000000000000000, -5.803681084894614095 ) ) ;
#27670=CYLINDRICAL_SURFACE ( 'NONE', #69039, 5.000000000000004441 ) ;
#27699=ADVANCED_FACE ( 'NONE', ( #760 ), #65131, .T. ) ;
#27768=VERTEX_POINT ( 'NONE', #23616 ) ;
#27827=CARTESIAN_POINT ( 'NONE',  ( 113.7642062731436141, 21.75126402171896345, -3.307110067226746608 ) ) ;
#27935=FACE_OUTER_BOUND ( 'NONE', #45959, .T. ) ;
#28117=ORIENTED_EDGE ( 'NONE', *, *, #44658, .T. ) ;
#28164=CARTESIAN_POINT ( 'NONE',  ( 110.6583185015671944, 21.43197767180794244, 4.967364376802527737 ) ) ;
#28366=FACE_OUTER_BOUND ( 'NONE', #1285, .T. ) ;
#28611=DIRECTION ( 'NONE',  ( 1.000000000000000000, 0.000000000000000000, 0.000000000000000000 ) ) ;
#28647=CARTESIAN_POINT ( 'NONE',  ( 280.0000000000000000, -21.42428528562853529, -4.999999999999990230 ) ) ;
#28653=CARTESIAN_POINT ( 'NONE',  ( 100.0000000000000284, 0.000000000000000000, 20.00000000000001421 ) ) ;
#28658=CARTESIAN_POINT ( 'NONE',  ( 276.6972452105824800, 21.67615690170940468, -3.768214559138908015 ) ) ;
#28685=EDGE_CURVE ( 'NONE', #64974, #27768, #24289, .T. ) ;
#28725=CARTESIAN_POINT ( 'NONE',  ( 107.7808008216759390, -21.53681828009572286, -4.492424461587423146 ) ) ;
#28726=DIRECTION ( 'NONE',  ( -1.000000000000000000, -0.000000000000000000, -0.000000000000000000 ) ) ;
#28753=ADVANCED_FACE ( 'NONE', ( #52589 ), #4070, .F. ) ;
#28917=DIRECTION ( 'NONE',  ( -0.000000000000000000, 1.000000000000000000, -0.000000000000000000 ) ) ;
#28940=CARTESIAN_POINT ( 'NONE',  ( 290.0000000000000568, 0.000000000000000000, 0.000000000000000000 ) ) ;
#28985=CIRCLE ( 'NONE', #46946, 20.00000000000001066 ) ;
#29008=CARTESIAN_POINT ( 'NONE',  ( 275.0002060648038196, -21.99995316709852133, 0.3345430166890087653 ) ) ;
#29019=CARTESIAN_POINT ( 'NONE',  ( 275.5071502593006585, 21.88997039781574472, 2.218170224452117978 ) ) ;
#29305=AXIS2_PLACEMENT_3D ( 'NONE', #39586, #14244, #67034 ) ;
#29337=CARTESIAN_POINT ( 'NONE',  ( 276.9490892766210663, -21.63874093657135589, -3.974828052515721577 ) ) ;
#29345=CARTESIAN_POINT ( 'NONE',  ( 278.3839814017205185, 21.48303375171747120, 4.742972355882017155 ) ) ;
#29377=FACE_BOUND ( 'NONE', #12409, .T. ) ;
#29426=CARTESIAN_POINT ( 'NONE',  ( 284.4930355657062364, -21.89000795769331731, -2.217852339353765245 ) ) ;
#29576=CARTESIAN_POINT ( 'NONE',  ( 55.00000000000000000, 0.000000000000000000, 0.000000000000000000 ) ) ;
#29607=VERTEX_POINT ( 'NONE', #32530 ) ;
#29682=CARTESIAN_POINT ( 'NONE',  ( 275.6635180218175947, -21.85802590693743852, 2.510273771313272562 ) ) ;
#29727=EDGE_CURVE ( 'NONE', #35721, #37319, #41105, .T. ) ;
#29764=ORIENTED_EDGE ( 'NONE', *, *, #60020, .F. ) ;
#29841=FACE_OUTER_BOUND ( 'NONE', #1329, .T. ) ;
#29880=CARTESIAN_POINT ( 'NONE',  ( -6.123233995736762338E-16, 0.000000000000000000, -20.00000000000000000 ) ) ;
#30036=CARTESIAN_POINT ( 'NONE',  ( 275.0322429538348956, -21.99260513325770106, -0.6553719608280085263 ) ) ;
#30046=CARTESIAN_POINT ( 'NONE',  ( 275.0320943261245361, 21.99263847259265958, 0.6545153999150201685 ) ) ;
#30192=EDGE_CURVE ( 'NONE', #1555, #44224, #38541, .T. ) ;
#30224=EDGE_CURVE ( 'NONE', #19726, #54877, #64801, .T. ) ;
#30306=CARTESIAN_POINT ( 'NONE',  ( 113.3057637310466532, -21.67663200833031922, -3.765392563550230332 ) ) ;
#30339=VERTEX_POINT ( 'NONE', #40842 ) ;
#30379=CARTESIAN_POINT ( 'NONE',  ( 107.4922189950060982, 21.56887920590508045, 4.337924292484288458 ) ) ;
#30430=DIRECTION ( 'NONE',  ( -0.000000000000000000, -0.000000000000000000, 1.000000000000000000 ) ) ;
#30450=CARTESIAN_POINT ( 'NONE',  ( 105.6635180218176231, -21.85802590693743852, 2.510273771313294322 ) ) ;
#30506=AXIS2_PLACEMENT_3D ( 'NONE', #20375, #3866, #41154 ) ;
#30579=EDGE_CURVE ( 'NONE', #25409, #8739, #49917, .T. ) ;
#30604=AXIS2_PLACEMENT_3D ( 'NONE', #29880, #62587, #41475 ) ;
#30718=VECTOR ( 'NONE', #51501, 1000.000000000000000 ) ;
#30723=CARTESIAN_POINT ( 'NONE',  ( 280.6524747721059612, 21.43176909745611169, -4.968265989321519527 ) ) ;
#30745=VERTEX_POINT ( 'NONE', #61529 ) ;
#30774=ORIENTED_EDGE ( 'NONE', *, *, #2544, .F. ) ;
#30801=CARTESIAN_POINT ( 'NONE',  ( 107.4947172190871356, -21.56856595115425890, 4.339532581985756643 ) ) ;
#30917=AXIS2_PLACEMENT_3D ( 'NONE', #58175, #52878, #63804 ) ;
#30978=CARTESIAN_POINT ( 'NONE',  ( 0.000000000000000000, 2.449293598294706907E-15, -20.00000000000000355 ) ) ;
#30999=CARTESIAN_POINT ( 'NONE',  ( 110.0000000000000284, -21.42428528562853529, 5.000000000000004441 ) ) ;
#31008=AXIS2_PLACEMENT_3D ( 'NONE', #38073, #38425, #47578 ) ;
#31342=CARTESIAN_POINT ( 'NONE',  ( 114.4935831913009565, -21.89011901571377194, 2.216886222927851868 ) ) ;
#31351=CARTESIAN_POINT ( 'NONE',  ( -1.224646799147352468E-15, 16.00000000000000000, 6.196318915105386793 ) ) ;
#31412=CARTESIAN_POINT ( 'NONE',  ( 282.2224082406586945, 21.53716320950900709, 4.490767689115649830 ) ) ;
#31418=CARTESIAN_POINT ( 'NONE',  ( 109.6730658560643974, 21.42428528562853174, -5.000000000000004441 ) ) ;
#31486=CARTESIAN_POINT ( 'NONE',  ( 105.2579562709429268, -21.94247096656776819, -1.618386763725522037 ) ) ;
#31677=EDGE_LOOP ( 'NONE', ( #6624, #46055, #25319, #50375, #9451 ) ) ;
#31686=EDGE_LOOP ( 'NONE', ( #66007, #48105, #66395, #25610 ) ) ;
#31763=CARTESIAN_POINT ( 'NONE',  ( 280.0000000000000000, -22.00000000000000000, -4.999999999999990230 ) ) ;
#31823=VERTEX_POINT ( 'NONE', #62925 ) ;
#31878=APPLICATION_CONTEXT ( 'automotive_design' ) ;
#31900=AXIS2_PLACEMENT_3D ( 'NONE', #24753, #46188, #57106 ) ;
#31932=CARTESIAN_POINT ( 'NONE',  ( 280.6598192889778716, -21.43204465433285932, 4.967071677942358932 ) ) ;
#32008=DIRECTION ( 'NONE',  ( -1.000000000000000000, -0.000000000000000000, -0.000000000000000000 ) ) ;
#32049=( GEOMETRIC_REPRESENTATION_CONTEXT ( 3 ) GLOBAL_UNCERTAINTY_ASSIGNED_CONTEXT ( ( #19115 ) ) GLOBAL_UNIT_ASSIGNED_CONTEXT ( ( #9698, #13930, #62468 ) ) REPRESENTATION_CONTEXT ( 'NONE', 'WORKASPACE' ) );
#32151=CARTESIAN_POINT ( 'NONE',  ( 100.0000000000000284, 2.449293598294708091E-15, -20.00000000000001421 ) ) ;
#32241=FACE_OUTER_BOUND ( 'NONE', #7811, .T. ) ;
#32246=VECTOR ( 'NONE', #24247, 1000.000000000000000 ) ;
#32279=CARTESIAN_POINT ( 'NONE',  ( 282.5114001799272501, -21.56931564127029688, 4.335727404899786919 ) ) ;
#32317=CYLINDRICAL_SURFACE ( 'NONE', #56455, 20.00000000000000355 ) ;
#32325=ORIENTED_EDGE ( 'NONE', *, *, #68737, .F. ) ;
#32445=CARTESIAN_POINT ( 'NONE',  ( 284.3399910931246950, 21.85871988289598988, 2.504349266409120478 ) ) ;
#32530=CARTESIAN_POINT ( 'NONE',  ( 55.00000000000000000, 16.00000000000000000, 6.196318915105386793 ) ) ;
#32581=DIRECTION ( 'NONE',  ( 1.000000000000000000, 0.000000000000000000, 0.000000000000000000 ) ) ;
#32588=DIRECTION ( 'NONE',  ( -0.000000000000000000, 1.000000000000000000, -0.000000000000000000 ) ) ;
#32598=EDGE_LOOP ( 'NONE', ( #64789, #23653, #2553, #36459 ) ) ;
#32985=PLANE ( 'NONE',  #35957 ) ;
#33091=CARTESIAN_POINT ( 'NONE',  ( 280.0000000000000000, 21.42428528562853529, 4.999999999999990230 ) ) ;
#33110=CARTESIAN_POINT ( 'NONE',  ( 114.4903733860909654, 21.88945422885941028, -2.223679814509753161 ) ) ;
#33259=DIRECTION ( 'NONE',  ( 0.000000000000000000, 0.000000000000000000, 1.000000000000000000 ) ) ;
#33399=ORIENTED_EDGE ( 'NONE', *, *, #36290, .T. ) ;
#33474=CARTESIAN_POINT ( 'NONE',  ( 113.7669346082183495, 21.75174821959686255, 3.303877464828373078 ) ) ;
#33518=CARTESIAN_POINT ( 'NONE',  ( -1.224646799147352468E-15, 16.00000000000000000, 6.196318915105386793 ) ) ;
#33525=ADVANCED_FACE ( 'NONE', ( #16302 ), #59540, .F. ) ;
#33605=EDGE_LOOP ( 'NONE', ( #12992, #1256, #46559, #44480, #63874, #5723 ) ) ;
#33608=EDGE_CURVE ( 'NONE', #13157, #25409, #68491, .T. ) ;
#33807=CARTESIAN_POINT ( 'NONE',  ( 114.9668435325539235, 21.99239968880144502, -0.6609596067687202314 ) ) ;
#33824=CARTESIAN_POINT ( 'NONE',  ( -1.224646799147352468E-15, 16.00000000000000000, 6.196318915105386793 ) ) ;
#33828=DIRECTION ( 'NONE',  ( -1.000000000000000000, -0.000000000000000000, -0.000000000000000000 ) ) ;
#33878=( LENGTH_UNIT ( ) NAMED_UNIT ( * ) SI_UNIT ( .MILLI., .METRE. ) );
#33939=CARTESIAN_POINT ( 'NONE',  ( 277.7789859651024358, 21.53699436807884027, 4.491592093615985881 ) ) ;
#34122=DIRECTION ( 'NONE',  ( -0.000000000000000000, 0.000000000000000000, 1.000000000000000000 ) ) ;
#34192=AXIS2_PLACEMENT_3D ( 'NONE', #15084, #10833, #69566 ) ;
#34229=SURFACE_STYLE_USAGE ( .BOTH. , #51096 ) ;
#34339=DIRECTION ( 'NONE',  ( -1.000000000000000000, -0.000000000000000000, -0.000000000000000000 ) ) ;
#34361=CARTESIAN_POINT ( 'NONE',  ( 106.6944765335652647, -21.67660392622676824, -3.765493530430633395 ) ) ;
#34529=CARTESIAN_POINT ( 'NONE',  ( 0.000000000000000000, 0.000000000000000000, 18.50000000000000000 ) ) ;
#34647=CARTESIAN_POINT ( 'NONE',  ( 276.9485791615414314, 21.63883785544751603, -3.974247539526118533 ) ) ;
#34812=CARTESIAN_POINT ( 'NONE',  ( -1.224646799147352468E-15, 16.00000000000000000, 6.196318915105386793 ) ) ;
#34818=DIRECTION ( 'NONE',  ( -1.000000000000000000, -0.000000000000000000, -0.000000000000000000 ) ) ;
#34965=CARTESIAN_POINT ( 'NONE',  ( 283.3030319151914682, 21.67621409537481014, -3.767785295203601059 ) ) ;
#34968=CARTESIAN_POINT ( 'NONE',  ( 277.4947172190871925, -21.56856595115426600, 4.339532581985733550 ) ) ;
#34976=CARTESIAN_POINT ( 'NONE',  ( 277.4892320395364322, 21.56923944770097279, -4.336110802034249367 ) ) ;
#35024=VECTOR ( 'NONE', #2193, 1000.000000000000000 ) ;
#35073=CARTESIAN_POINT ( 'NONE',  ( 100.0000000000000284, 5.000000000000000000, 18.50000000000000000 ) ) ;
#35312=CARTESIAN_POINT ( 'NONE',  ( 105.5071502593007722, 21.88997039781574472, 2.218170224452124195 ) ) ;
#35318=CARTESIAN_POINT ( 'NONE',  ( 279.6684666882774195, 21.42428528562853174, 4.999999999999991118 ) ) ;
#35331=EDGE_CURVE ( 'NONE', #35721, #60501, #48336, .T. ) ;
#35457=ORIENTED_EDGE ( 'NONE', *, *, #33608, .T. ) ;
#35610=PRODUCT_DEFINITION_SHAPE ( 'NONE', 'NONE',  #43475 ) ;
#35657=CARTESIAN_POINT ( 'NONE',  ( 284.4903733860909938, 21.88945422885941028, -2.223679814509739394 ) ) ;
#35672=VECTOR ( 'NONE', #6667, 1000.000000000000000 ) ;
#35721=VERTEX_POINT ( 'NONE', #8298 ) ;
#35749=CARTESIAN_POINT ( 'NONE',  ( 100.0000000000000284, 5.000000000000000000, 18.50000000000000000 ) ) ;
#35957=AXIS2_PLACEMENT_3D ( 'NONE', #31351, #20432, #10222 ) ;
#35982=AXIS2_PLACEMENT_3D ( 'NONE', #13997, #40380, #3443 ) ;
#35994=UNCERTAINTY_MEASURE_WITH_UNIT (LENGTH_MEASURE( 1.000000000000000082E-05 ), #33878, 'distance_accuracy_value', 'NONE');
#36075=CARTESIAN_POINT ( 'NONE',  ( 105.5096892522198573, -21.88944388124440721, 2.223599993928985885 ) ) ;
#36290=EDGE_CURVE ( 'NONE', #18523, #54877, #65318, .T. ) ;
#36349=CARTESIAN_POINT ( 'NONE',  ( 108.7021502624939302, 21.46117544541992572, 4.839652729015487154 ) ) ;
#36429=CIRCLE ( 'NONE', #3846, 20.00000000000000355 ) ;
#36459=ORIENTED_EDGE ( 'NONE', *, *, #38007, .F. ) ;
#36520=ORIENTED_EDGE ( 'NONE', *, *, #5320, .F. ) ;
#36521=VECTOR ( 'NONE', #15541, 1000.000000000000000 ) ;
#36621=CARTESIAN_POINT ( 'NONE',  ( 114.4930355657061511, -21.89000795769331376, -2.217852339353778124 ) ) ;
#36695=DIRECTION ( 'NONE',  ( -0.000000000000000000, 1.000000000000000000, -0.000000000000000000 ) ) ;
#36701=CARTESIAN_POINT ( 'NONE',  ( 107.4892320395363186, 21.56923944770097634, -4.336110802034259137 ) ) ;
#36769=CARTESIAN_POINT ( 'NONE',  ( 105.1608565259479633, -21.96391085485758410, -1.300312621757638620 ) ) ;
#37145=EDGE_CURVE ( 'NONE', #11779, #13157, #23727, .T. ) ;
#37299=EDGE_CURVE ( 'NONE', #44224, #1555, #20069, .T. ) ;
#37319=VERTEX_POINT ( 'NONE', #19132 ) ;
#37345=CARTESIAN_POINT ( 'NONE',  ( 290.0000000000000568, -5.000000000000000888, 21.42428528562853529 ) ) ;
#37357=CARTESIAN_POINT ( 'NONE',  ( 284.9679224117287504, 21.99264416388322374, 0.6532133356533497137 ) ) ;
#37365=CARTESIAN_POINT ( 'NONE',  ( 106.9485791615413461, 21.63883785544751603, -3.974247539526119422 ) ) ;
#37479=VECTOR ( 'NONE', #62644, 1000.000000000000000 ) ;
#37502=PLANE ( 'NONE',  #12295 ) ;
#37538=EDGE_CURVE ( 'NONE', #39848, #1555, #63784, .T. ) ;
#37614=CARTESIAN_POINT ( 'NONE',  ( 100.0000000000000284, 0.000000000000000000, 0.000000000000000000 ) ) ;
#37680=CARTESIAN_POINT ( 'NONE',  ( 114.9679224117287646, 21.99264416388322374, 0.6532133356533591506 ) ) ;
#37703=AXIS2_PLACEMENT_3D ( 'NONE', #19170, #56117, #17798 ) ;
#37730=EDGE_CURVE ( 'NONE', #42114, #35721, #7112, .T. ) ;
#37846=DIRECTION ( 'NONE',  ( 0.000000000000000000, -0.000000000000000000, 1.000000000000000000 ) ) ;
#38007=EDGE_CURVE ( 'NONE', #27768, #19247, #21463, .T. ) ;
#38073=CARTESIAN_POINT ( 'NONE',  ( 290.0000000000000568, 0.000000000000000000, 0.000000000000000000 ) ) ;
#38109=CARTESIAN_POINT ( 'NONE',  ( 290.0000000000000568, 0.000000000000000000, 19.99999999999998934 ) ) ;
#38187=DIRECTION ( 'NONE',  ( 0.000000000000000000, 1.000000000000000000, 0.000000000000000000 ) ) ;
#38199=CARTESIAN_POINT ( 'NONE',  ( -1.224646799147352468E-15, 0.000000000000000000, 0.000000000000000000 ) ) ;
#38202=ADVANCED_FACE ( 'NONE', ( #12661 ), #40086, .F. ) ;
#38210=ADVANCED_FACE ( 'NONE', ( #45358 ), #12312, .T. ) ;
#38234=CARTESIAN_POINT ( 'NONE',  ( 283.7689755057785987, -21.75207715352313542, 3.301879156304023510 ) ) ;
#38270=FACE_OUTER_BOUND ( 'NONE', #31677, .T. ) ;
#38344=ADVANCED_FACE ( 'NONE', ( #4184 ), #46047, .F. ) ;
#38425=DIRECTION ( 'NONE',  ( -1.000000000000000000, -0.000000000000000000, -0.000000000000000000 ) ) ;
#38541=B_SPLINE_CURVE_WITH_KNOTS ( 'NONE', 3,
 ( #57449, #68359, #30723, #19466, #14199, #25798, #61685, #13509, #34965, #56408, #56762, #8584, #35657, #57112, #8925, #47914, #54219, #53183, #37357, #9959, #42648, #10627, #32445, #43323, #4664, #426, #53874, #11318, #31412, #5012, #15582, #52842, #58141, #58816 ),
 .UNSPECIFIED., .F., .F.,
 ( 4, 2, 2, 2, 2, 2, 2, 2, 2, 2, 2, 2, 2, 2, 2, 2, 4 ),
 ( 0.01568356594869772802, 0.01666352729433782584, 0.01764348863997792019, 0.01862344998561801801, 0.01960341133125811236, 0.02058337267689821018, 0.02156333402253830800, 0.02254329536817840235, 0.02352325671381850017, 0.02450321805945859799, 0.02548317940509869234, 0.02646314075073879016, 0.02744310209637888798, 0.02842306344201898233, 0.02940302478765908015, 0.03038298613329917797, 0.03136294747893927232 ),
 .UNSPECIFIED. ) ;
#38639=CIRCLE ( 'NONE', #12799, 20.00000000000001066 ) ;
#38723=ORIENTED_EDGE ( 'NONE', *, *, #28685, .T. ) ;
#38768=EDGE_LOOP ( 'NONE', ( #54195, #59206, #698, #32325 ) ) ;
#38857=DIRECTION ( 'NONE',  ( 0.000000000000000000, 0.000000000000000000, -1.000000000000000000 ) ) ;
#38950=CARTESIAN_POINT ( 'NONE',  ( 282.5087422071486571, -21.56900326173647997, -4.337278505387078376 ) ) ;
#39052=DIRECTION ( 'NONE',  ( -1.000000000000000000, 0.000000000000000000, -0.000000000000000000 ) ) ;
#39095=CARTESIAN_POINT ( 'NONE',  ( 114.8388692023054318, 21.96385131419673442, -1.300671796277839354 ) ) ;
#39174=DIRECTION ( 'NONE',  ( -1.000000000000000000, -0.000000000000000000, -0.000000000000000000 ) ) ;
#39206=CARTESIAN_POINT ( 'NONE',  ( 279.3447482101068431, -21.43190799616912656, -4.967656235065410542 ) ) ;
#39356=PLANE ( 'NONE',  #25313 ) ;
#39484=ORIENTED_EDGE ( 'NONE', *, *, #11120, .T. ) ;
#39509=ORIENTED_EDGE ( 'NONE', *, *, #61693, .F. ) ;
#39542=ORIENTED_EDGE ( 'NONE', *, *, #63706, .T. ) ;
#39586=CARTESIAN_POINT ( 'NONE',  ( 0.000000000000000000, 0.000000000000000000, 0.000000000000000000 ) ) ;
#39804=CIRCLE ( 'NONE', #34192, 20.00000000000000000 ) ;
#39848=VERTEX_POINT ( 'NONE', #3884 ) ;
#39892=CARTESIAN_POINT ( 'NONE',  ( 275.1611065714564575, -21.96385652020510193, 1.300672318859845911 ) ) ;
#39902=CARTESIAN_POINT ( 'NONE',  ( 276.0251321087873180, 21.78917327468806420, -3.050596224313125493 ) ) ;
#39979=CARTESIAN_POINT ( 'NONE',  ( 284.3366190915103857, -21.85805078441903504, -2.510101233139093502 ) ) ;
#40017=B_SPLINE_CURVE_WITH_KNOTS ( 'NONE', 3,
 ( #16085, #10458, #31932, #65325, #10811, #43502, #32279, #16775, #5532, #38234, #6220, #50186, #56154, #44194, #17834, #45600, #49469, #1304, #7971, #22755, #44908, #29426, #39979, #2695, #50876, #54753, #61438, #38950, #24159, #66041, #65681, #7638, #67086, #55102 ),
 .UNSPECIFIED., .F., .F.,
 ( 4, 2, 2, 2, 2, 2, 2, 2, 2, 2, 2, 2, 2, 2, 2, 2, 4 ),
 ( 0.007843851441979901237, 0.008823947846603227146, 0.009804044251226553056, 0.01078414065584987896, 0.01176423706047320487, 0.01274433346509653078, 0.01372442986971985669, 0.01470452627434318260, 0.01568462267896651025, 0.01666471908358983442, 0.01764481548821315859, 0.01862491189283648624, 0.01960500829745981388, 0.02058510470208313806, 0.02156520110670646223, 0.02254529751132978987, 0.02352539391595311752 ),
 .UNSPECIFIED. ) ;
#40086=PLANE ( 'NONE',  #45207 ) ;
#40244=CARTESIAN_POINT ( 'NONE',  ( 277.4937869665631069, -21.56868463414005177, -4.338918127843128580 ) ) ;
#40251=CARTESIAN_POINT ( 'NONE',  ( 275.0001309909290512, 21.99997022933651891, 0.3293293811575784269 ) ) ;
#40380=DIRECTION ( 'NONE',  ( -1.000000000000000000, -0.000000000000000000, -0.000000000000000000 ) ) ;
#40388=ORIENTED_EDGE ( 'NONE', *, *, #41395, .T. ) ;
#40423=AXIS2_PLACEMENT_3D ( 'NONE', #26857, #48283, #5735 ) ;
#40782=CARTESIAN_POINT ( 'NONE',  ( -2.282530889443167084E-17, -4.999999999999999112, 21.42428528562853529 ) ) ;
#40827=ORIENTED_EDGE ( 'NONE', *, *, #60282, .F. ) ;
#40842=CARTESIAN_POINT ( 'NONE',  ( -1.224646799147352468E-15, 2.449293598294706513E-15, -20.00000000000000000 ) ) ;
#40991=B_SPLINE_CURVE_WITH_KNOTS ( 'NONE', 3,
 ( #30999, #3915, #41546, #24688, #53114, #67947, #62664, #20775, #47491, #52447, #25034, #25727, #31342, #68288, #26064, #20093, #46467, #15160, #47156, #63001, #68620, #36621, #19742, #19392, #41205, #30306, #20425, #41889, #63349, #58071, #4598, #68952, #14472, #42237 ),
 .UNSPECIFIED., .F., .F.,
 ( 4, 2, 2, 2, 2, 2, 2, 2, 2, 2, 2, 2, 2, 2, 2, 2, 4 ),
 ( 0.007843851441979916850, 0.008823947846603241024, 0.009804044251226563464, 0.01078414065584988764, 0.01176423706047321008, 0.01274433346509653425, 0.01372442986971985843, 0.01470452627434318260, 0.01568462267896650331, 0.01666471908358983095, 0.01764481548821315166, 0.01862491189283647583, 0.01960500829745980000, 0.02058510470208312071, 0.02156520110670644835, 0.02254529751132976906, 0.02352539391595309323 ),
 .UNSPECIFIED. ) ;
#41009=CARTESIAN_POINT ( 'NONE',  ( 106.9483136162804584, -21.63883973695288887, 3.974316929722046865 ) ) ;
#41045=DIRECTION ( 'NONE',  ( -1.000000000000000000, -4.565061778886334783E-18, -0.000000000000000000 ) ) ;
#41061=EDGE_CURVE ( 'NONE', #29607, #17632, #49113, .T. ) ;
#41105=LINE ( 'NONE', #50966, #32246 ) ;
#41154=DIRECTION ( 'NONE',  ( 0.000000000000000000, 0.000000000000000000, 1.000000000000000000 ) ) ;
#41193=VECTOR ( 'NONE', #22951, 1000.000000000000000 ) ;
#41205=CARTESIAN_POINT ( 'NONE',  ( 113.7666631852362542, -21.75169080623576079, -3.304315882619072831 ) ) ;
#41283=CARTESIAN_POINT ( 'NONE',  ( 106.0273295991593301, 21.78875652052166956, 3.053836096979983594 ) ) ;
#41316=ORIENTED_EDGE ( 'NONE', *, *, #68737, .T. ) ;
#41395=EDGE_CURVE ( 'NONE', #6688, #3562, #7189, .T. ) ;
#41475=DIRECTION ( 'NONE',  ( 0.000000000000000000, 0.000000000000000000, -1.000000000000000000 ) ) ;
#41546=CARTESIAN_POINT ( 'NONE',  ( 110.6598192889778574, -21.43204465433285932, 4.967071677942377583 ) ) ;
#41648=VECTOR ( 'NONE', #5862, 1000.000000000000000 ) ;
#41694=CARTESIAN_POINT ( 'NONE',  ( 105.0322429538348672, -21.99260513325770816, -0.6553719608279887643 ) ) ;
#41889=CARTESIAN_POINT ( 'NONE',  ( 112.5087422071486856, -21.56900326173646931, -4.337278505387113015 ) ) ;
#41936=ORIENTED_EDGE ( 'NONE', *, *, #61693, .T. ) ;
#42037=CARTESIAN_POINT ( 'NONE',  ( 105.5080822241900762, -21.88977794987918557, -2.220096651196666659 ) ) ;
#42114=VERTEX_POINT ( 'NONE', #10575 ) ;
#42237=CARTESIAN_POINT ( 'NONE',  ( 110.0000000000000284, -21.42428528562853174, -5.000000000000004441 ) ) ;
#42314=CARTESIAN_POINT ( 'NONE',  ( 106.6972452105824800, 21.67615690170939757, -3.768214559138922226 ) ) ;
#42323=CARTESIAN_POINT ( 'NONE',  ( 290.0000000000000568, -5.000000000000000888, 19.36491673103706290 ) ) ;
#42398=CIRCLE ( 'NONE', #68221, 20.00000000000001066 ) ;
#42444=ORIENTED_EDGE ( 'NONE', *, *, #20573, .T. ) ;
#42551=ORIENTED_EDGE ( 'NONE', *, *, #30192, .T. ) ;
#42644=ADVANCED_FACE ( 'NONE', ( #43112 ), #64581, .T. ) ;
#42648=CARTESIAN_POINT ( 'NONE',  ( 284.7436796776308938, 21.94282408638629889, 1.613761426918498776 ) ) ;
#42654=CARTESIAN_POINT ( 'NONE',  ( 105.1286806118793749, 21.97108935923501960, 1.139020068845009614 ) ) ;
#42841=ORIENTED_EDGE ( 'NONE', *, *, #57039, .F. ) ;
#42907=CARTESIAN_POINT ( 'NONE',  ( 110.0000000000000284, -22.00000000000000000, 5.000000000000004441 ) ) ;
#42930=FACE_OUTER_BOUND ( 'NONE', #56166, .T. ) ;
#42946=CARTESIAN_POINT ( 'NONE',  ( 111.3012118866375033, 21.46131765974229566, -4.839032743736826347 ) ) ;
#43020=EDGE_LOOP ( 'NONE', ( #40827, #20767, #11775, #39542, #57360 ) ) ;
#43021=ORIENTED_EDGE ( 'NONE', *, *, #41061, .F. ) ;
#43056=APPLICATION_CONTEXT ( 'automotive_design' ) ;
#43112=FACE_OUTER_BOUND ( 'NONE', #20355, .T. ) ;
#43183=AXIS2_PLACEMENT_3D ( 'NONE', #28940, #806, #60239 ) ;
#43274=CARTESIAN_POINT ( 'NONE',  ( 290.0000000000000568, -5.000000000000000888, 18.50000000000000000 ) ) ;
#43323=CARTESIAN_POINT ( 'NONE',  ( 283.9761838721219078, 21.78940454476515853, 3.049139182071509691 ) ) ;
#43399=DIRECTION ( 'NONE',  ( -0.000000000000000000, 1.000000000000000000, -0.000000000000000000 ) ) ;
#43411=CARTESIAN_POINT ( 'NONE',  ( 100.0000000000000284, 0.000000000000000000, 0.000000000000000000 ) ) ;
#43475=PRODUCT_DEFINITION ( 'UNKNOWN', '', #4140, #778 ) ;
#43501=EDGE_CURVE ( 'NONE', #54597, #11779, #4391, .T. ) ;
#43502=CARTESIAN_POINT ( 'NONE',  ( 282.2205320413087293, -21.53693364843037017, 4.491889980468770638 ) ) ;
#43548=ORIENTED_EDGE ( 'NONE', *, *, #3905, .T. ) ;
#43625=LINE ( 'NONE', #43274, #23332 ) ;
#43672=VECTOR ( 'NONE', #60831, 1000.000000000000000 ) ;
#43691=FACE_OUTER_BOUND ( 'NONE', #48492, .T. ) ;
#43767=CARTESIAN_POINT ( 'NONE',  ( 290.0000000000000568, 0.000000000000000000, 0.000000000000000000 ) ) ;
#43815=EDGE_CURVE ( 'NONE', #42114, #59695, #54900, .T. ) ;
#44077=ORIENTED_EDGE ( 'NONE', *, *, #10930, .T. ) ;
#44194=CARTESIAN_POINT ( 'NONE',  ( 284.7439874972685061, -21.94289037477085813, 1.612903297879183961 ) ) ;
#44214=ADVANCED_FACE ( 'NONE', ( #42930 ), #15866, .F. ) ;
#44224=VERTEX_POINT ( 'NONE', #33091 ) ;
#44300=ORIENTED_EDGE ( 'NONE', *, *, #60020, .T. ) ;
#44346=CARTESIAN_POINT ( 'NONE',  ( 112.5088088673474687, 21.56899521162237576, -4.337361123092376758 ) ) ;
#44385=AXIS2_PLACEMENT_3D ( 'NONE', #63375, #27105, #53136 ) ;
#44480=ORIENTED_EDGE ( 'NONE', *, *, #43501, .T. ) ;
#44529=DIRECTION ( 'NONE',  ( 0.000000000000000000, 0.000000000000000000, 1.000000000000000000 ) ) ;
#44552=CARTESIAN_POINT ( 'NONE',  ( 0.000000000000000000, 0.000000000000000000, 0.000000000000000000 ) ) ;
#44558=DIRECTION ( 'NONE',  ( 0.000000000000000000, 0.000000000000000000, 1.000000000000000000 ) ) ;
#44658=EDGE_CURVE ( 'NONE', #30339, #30745, #63525, .T. ) ;
#44833=CARTESIAN_POINT ( 'NONE',  ( 275.3198800741404284, 21.92942769035742145, 1.767193244627905946 ) ) ;
#44863=EDGE_LOOP ( 'NONE', ( #13991, #14334, #57171, #35457, #63364 ) ) ;
#44908=CARTESIAN_POINT ( 'NONE',  ( 284.7429429236411806, -21.94266591301279234, -1.615775360921237747 ) ) ;
#44952=CARTESIAN_POINT ( 'NONE',  ( 100.0000000000000284, 5.000000000000002665, 19.36491673103709488 ) ) ;
#45015=VERTEX_POINT ( 'NONE', #38109 ) ;
#45063=VERTEX_POINT ( 'NONE', #32151 ) ;
#45173=CARTESIAN_POINT ( 'NONE',  ( 275.6617573822855434, 21.85836566642199230, 2.507523880400401417 ) ) ;
#45207=AXIS2_PLACEMENT_3D ( 'NONE', #50987, #39052, #34122 ) ;
#45238=CARTESIAN_POINT ( 'NONE',  ( 110.0000000000000284, -21.42428528562853174, -5.000000000000004441 ) ) ;
#45358=FACE_OUTER_BOUND ( 'NONE', #43020, .T. ) ;
#45469=ORIENTED_EDGE ( 'NONE', *, *, #18507, .F. ) ;
#45472=CARTESIAN_POINT ( 'NONE',  ( 100.0000000000000284, 0.000000000000000000, 0.000000000000000000 ) ) ;
#45494=ORIENTED_EDGE ( 'NONE', *, *, #960, .T. ) ;
#45511=CARTESIAN_POINT ( 'NONE',  ( 278.2349883415517411, -21.49634503089637150, 4.680941717099500465 ) ) ;
#45548=FACE_BOUND ( 'NONE', #25577, .T. ) ;
#45600=CARTESIAN_POINT ( 'NONE',  ( 284.9673805781174565, -21.99252023018708968, 0.6578219585122039303 ) ) ;
#45842=LINE ( 'NONE', #7870, #9364 ) ;
#45866=CARTESIAN_POINT ( 'NONE',  ( 106.6934359423128598, 21.67676124233545565, 3.764605836381888615 ) ) ;
#45870=VERTEX_POINT ( 'NONE', #6981 ) ;
#45882=ORIENTED_EDGE ( 'NONE', *, *, #51556, .T. ) ;
#45959=EDGE_LOOP ( 'NONE', ( #1903, #23848, #7649, #59670, #27474 ) ) ;
#46047=PLANE ( 'NONE',  #30604 ) ;
#46055=ORIENTED_EDGE ( 'NONE', *, *, #2544, .T. ) ;
#46188=DIRECTION ( 'NONE',  ( 1.000000000000000000, 0.000000000000000000, -0.000000000000000000 ) ) ;
#46194=CARTESIAN_POINT ( 'NONE',  ( 279.3475734619033233, -21.43178884250801630, 4.968175626252045340 ) ) ;
#46203=CARTESIAN_POINT ( 'NONE',  ( 275.6635354938838987, 21.85802876872917366, -2.510136981039510662 ) ) ;
#46266=VERTEX_POINT ( 'NONE', #15563 ) ;
#46467=CARTESIAN_POINT ( 'NONE',  ( 115.0000633975120365, -22.00001440852518897, 0.3259197091964680659 ) ) ;
#46520=ORIENTED_EDGE ( 'NONE', *, *, #29727, .T. ) ;
#46559=ORIENTED_EDGE ( 'NONE', *, *, #19324, .F. ) ;
#46623=CARTESIAN_POINT ( 'NONE',  ( 107.7840330814956786, -21.53650026154319264, 4.493931093091683593 ) ) ;
#46892=FACE_OUTER_BOUND ( 'NONE', #44863, .T. ) ;
#46946=AXIS2_PLACEMENT_3D ( 'NONE', #49755, #55751, #33259 ) ;
#46972=CARTESIAN_POINT ( 'NONE',  ( 105.1611065714564006, -21.96385652020509838, 1.300672318859854126 ) ) ;
#46997=EDGE_CURVE ( 'NONE', #47125, #31823, #54717, .T. ) ;
#47010=LINE ( 'NONE', #8352, #19304 ) ;
#47125=VERTEX_POINT ( 'NONE', #12544 ) ;
#47137=ORIENTED_EDGE ( 'NONE', *, *, #26604, .T. ) ;
#47156=CARTESIAN_POINT ( 'NONE',  ( 114.9681307937126320, -21.99268844340181417, -0.6535439379101506407 ) ) ;
#47174=ORIENTED_EDGE ( 'NONE', *, *, #10333, .T. ) ;
#47220=ADVANCED_FACE ( 'NONE', ( #28366 ), #23102, .T. ) ;
#47386=DIRECTION ( 'NONE',  ( -1.000000000000000000, -0.000000000000000000, -0.000000000000000000 ) ) ;
#47430=DIRECTION ( 'NONE',  ( -1.000000000000000000, -0.000000000000000000, -0.000000000000000000 ) ) ;
#47491=CARTESIAN_POINT ( 'NONE',  ( 113.3053295232375319, -21.67655155662104249, 3.765949955696211937 ) ) ;
#47522=LINE ( 'NONE', #9920, #36521 ) ;
#47560=CARTESIAN_POINT ( 'NONE',  ( 290.0000000000000568, 0.000000000000000000, -19.99999999999997868 ) ) ;
#47578=DIRECTION ( 'NONE',  ( 0.000000000000000000, 0.000000000000000000, 1.000000000000000000 ) ) ;
#47598=CYLINDRICAL_SURFACE ( 'NONE', #30917, 19.99999999999998934 ) ;
#47912=DIRECTION ( 'NONE',  ( -1.000000000000000000, 0.000000000000000000, -0.000000000000000000 ) ) ;
#47914=CARTESIAN_POINT ( 'NONE',  ( 284.9668435325538667, 21.99239968880144502, -0.6609596067687139032 ) ) ;
#48105=ORIENTED_EDGE ( 'NONE', *, *, #37538, .T. ) ;
#48124=ADVANCED_FACE ( 'NONE', ( #55630 ), #18703, .F. ) ;
#48217=CARTESIAN_POINT ( 'NONE',  ( 111.3030933484817382, 21.46146164524274980, 4.838392277045666212 ) ) ;
#48283=DIRECTION ( 'NONE',  ( -1.000000000000000000, -0.000000000000000000, -0.000000000000000000 ) ) ;
#48336=CIRCLE ( 'NONE', #35982, 20.00000000000001066 ) ;
#48492=EDGE_LOOP ( 'NONE', ( #64288, #49585, #11931, #66924, #46520, #42841 ) ) ;
#48628=CARTESIAN_POINT ( 'NONE',  ( 55.00000000000000000, 16.00000000000000000, -5.803681084894614095 ) ) ;
#48901=EDGE_LOOP ( 'NONE', ( #25868, #61650, #45494, #28117, #15569, #54819 ) ) ;
#48945=CARTESIAN_POINT ( 'NONE',  ( 106.0251321087872896, 21.78917327468806064, -3.050596224313125493 ) ) ;
#49027=CARTESIAN_POINT ( 'NONE',  ( 278.3842135503132340, -21.48302731199174787, -4.742990268296088274 ) ) ;
#49113=LINE ( 'NONE', #952, #67918 ) ;
#49397=EDGE_CURVE ( 'NONE', #27768, #64974, #40991, .T. ) ;
#49469=CARTESIAN_POINT ( 'NONE',  ( 285.0000633975121218, -22.00001440852518897, 0.3259197091964841642 ) ) ;
#49585=ORIENTED_EDGE ( 'NONE', *, *, #12554, .F. ) ;
#49586=ORIENTED_EDGE ( 'NONE', *, *, #25374, .T. ) ;
#49755=CARTESIAN_POINT ( 'NONE',  ( 100.0000000000000284, 0.000000000000000000, 0.000000000000000000 ) ) ;
#49777=VECTOR ( 'NONE', #43399, 1000.000000000000000 ) ;
#49917=LINE ( 'NONE', #60823, #35672 ) ;
#50050=FILL_AREA_STYLE ('',( #2560 ) ) ;
#50126=ORIENTED_EDGE ( 'NONE', *, *, #3905, .F. ) ;
#50174=CARTESIAN_POINT ( 'NONE',  ( 109.6700404598697958, -21.42428528562852819, -5.000000000000006217 ) ) ;
#50186=CARTESIAN_POINT ( 'NONE',  ( 284.3366674800922169, -21.85806848808613267, 2.509805449638021990 ) ) ;
#50272=EDGE_CURVE ( 'NONE', #60501, #3562, #28985, .T. ) ;
#50375=ORIENTED_EDGE ( 'NONE', *, *, #19457, .T. ) ;
#50451=CARTESIAN_POINT ( 'NONE',  ( 275.2579562709427705, -21.94247096656777174, -1.618386763725532917 ) ) ;
#50459=CARTESIAN_POINT ( 'NONE',  ( 275.2647131865113010, 21.94130279673636608, 1.613668875657348512 ) ) ;
#50530=CARTESIAN_POINT ( 'NONE',  ( 0.000000000000000000, 0.000000000000000000, 0.000000000000000000 ) ) ;
#50695=LINE ( 'NONE', #18693, #8462 ) ;
#50734=VECTOR ( 'NONE', #41045, 1000.000000000000000 ) ;
#50767=DIRECTION ( 'NONE',  ( 0.000000000000000000, -1.000000000000000000, 0.000000000000000000 ) ) ;
#50789=CARTESIAN_POINT ( 'NONE',  ( 275.0330373230561349, -21.99242646597929252, 0.6602422734858162112 ) ) ;
#50799=CARTESIAN_POINT ( 'NONE',  ( 280.0000000000000000, 21.42428528562853884, -4.999999999999990230 ) ) ;
#50832=DIRECTION ( 'NONE',  ( -4.565061778886334783E-18, 1.000000000000000000, 0.000000000000000000 ) ) ;
#50856=ADVANCED_FACE ( 'NONE', ( #29377, #2648, #45548, #61724, #13549 ), #7589, .T. ) ;
#50876=CARTESIAN_POINT ( 'NONE',  ( 283.7666631852362116, -21.75169080623575724, -3.304315882619051514 ) ) ;
#50894=AXIS2_PLACEMENT_3D ( 'NONE', #43411, #64889, #60302 ) ;
#50942=CARTESIAN_POINT ( 'NONE',  ( 280.0000000000000000, 21.42428528562853884, -4.999999999999990230 ) ) ;
#50966=CARTESIAN_POINT ( 'NONE',  ( 100.0000000000000284, -5.000000000000000000, 18.50000000000000000 ) ) ;
#50987=CARTESIAN_POINT ( 'NONE',  ( 100.0000000000000284, 5.000000000000000000, 18.50000000000000000 ) ) ;
#50993=AXIS2_PLACEMENT_3D ( 'NONE', #47560, #47912, #26813 ) ;
#51003=EDGE_CURVE ( 'NONE', #7734, #68664, #54971, .T. ) ;
#51044=DIRECTION ( 'NONE',  ( 0.000000000000000000, 0.000000000000000000, -1.000000000000000000 ) ) ;
#51096=SURFACE_SIDE_STYLE ('',( #13121 ) ) ;
#51158=CARTESIAN_POINT ( 'NONE',  ( 275.1286806118793038, 21.97108935923501605, 1.139020068845007838 ) ) ;
#51311=CARTESIAN_POINT ( 'NONE',  ( -1.224646799147352468E-15, 16.00000000000000000, -5.803681084894614095 ) ) ;
#51499=CARTESIAN_POINT ( 'NONE',  ( 276.6971892993743154, -21.67618688890531686, 3.767895544566218113 ) ) ;
#51501=DIRECTION ( 'NONE',  ( -1.000000000000000000, -0.000000000000000000, -0.000000000000000000 ) ) ;
#51506=CARTESIAN_POINT ( 'NONE',  ( 274.9998698049113273, 22.00002958979062839, -0.3253397936367980470 ) ) ;
#51556=EDGE_CURVE ( 'NONE', #31823, #47125, #8012, .T. ) ;
#52366=ORIENTED_EDGE ( 'NONE', *, *, #53660, .T. ) ;
#52447=CARTESIAN_POINT ( 'NONE',  ( 113.7689755057786272, -21.75207715352313542, 3.301879156304019070 ) ) ;
#52589=FACE_OUTER_BOUND ( 'NONE', #32598, .T. ) ;
#52842=CARTESIAN_POINT ( 'NONE',  ( 280.6583185015672370, 21.43197767180794244, 4.967364376802513526 ) ) ;
#52878=DIRECTION ( 'NONE',  ( -1.000000000000000000, -0.000000000000000000, -0.000000000000000000 ) ) ;
#53114=CARTESIAN_POINT ( 'NONE',  ( 111.6139602183311155, -21.48286796535249721, 4.743729604094153451 ) ) ;
#53134=EDGE_LOOP ( 'NONE', ( #45882, #58791, #1629, #12659, #24053 ) ) ;
#53136=DIRECTION ( 'NONE',  ( -0.000000000000000000, 0.000000000000000000, 1.000000000000000000 ) ) ;
#53183=CARTESIAN_POINT ( 'NONE',  ( 285.0001299725262243, 22.00002953920830606, 0.3279435515783846178 ) ) ;
#53189=CARTESIAN_POINT ( 'NONE',  ( 105.0001309909291365, 21.99997022933652246, 0.3293293811575764285 ) ) ;
#53310=ORIENTED_EDGE ( 'NONE', *, *, #2005, .F. ) ;
#53330=LINE ( 'NONE', #5161, #8780 ) ;
#53412=CIRCLE ( 'NONE', #31008, 22.00000000000000000 ) ;
#53541=CARTESIAN_POINT ( 'NONE',  ( 105.0326735325357248, 21.99250842598269173, -0.6579281897535147472 ) ) ;
#53568=FACE_OUTER_BOUND ( 'NONE', #53134, .T. ) ;
#53587=CARTESIAN_POINT ( 'NONE',  ( -6.123233995736762338E-16, 16.00000000000000000, -5.803681084894614095 ) ) ;
#53641=EDGE_CURVE ( 'NONE', #11717, #37319, #56460, .T. ) ;
#53660=EDGE_CURVE ( 'NONE', #39848, #16987, #14427, .T. ) ;
#53675=CARTESIAN_POINT ( 'NONE',  ( 100.0000000000000284, 0.000000000000000000, -21.99999999999997158 ) ) ;
#53746=CARTESIAN_POINT ( 'NONE',  ( 0.000000000000000000, 0.000000000000000000, 0.000000000000000000 ) ) ;
#53766=ORIENTED_EDGE ( 'NONE', *, *, #53641, .T. ) ;
#53844=CARTESIAN_POINT ( 'NONE',  ( 114.8405205227988546, 21.96421596965998901, 1.294720749503662116 ) ) ;
#53874=CARTESIAN_POINT ( 'NONE',  ( 283.0554507864566176, 21.63937313260594664, 3.971423903130205879 ) ) ;
#53880=CARTESIAN_POINT ( 'NONE',  ( 106.2331853604024587, 21.75170065437620437, -3.304351318131959925 ) ) ;
#53933=EDGE_LOOP ( 'NONE', ( #43021, #39509, #10637, #50126 ) ) ;
#54036=CARTESIAN_POINT ( 'NONE',  ( 0.000000000000000000, 19.13941707223176181, -5.803681084894614095 ) ) ;
#54037=FACE_OUTER_BOUND ( 'NONE', #12521, .T. ) ;
#54066=VECTOR ( 'NONE', #16188, 1000.000000000000000 ) ;
#54195=ORIENTED_EDGE ( 'NONE', *, *, #30224, .F. ) ;
#54219=CARTESIAN_POINT ( 'NONE',  ( 284.9998692468128638, 21.99997028336874294, -0.3318949079940898828 ) ) ;
#54546=CARTESIAN_POINT ( 'NONE',  ( 113.9746407525165779, 21.78913134333903301, -3.050900938606327273 ) ) ;
#54597=VERTEX_POINT ( 'NONE', #12835 ) ;
#54599=DIRECTION ( 'NONE',  ( -4.565061778886334783E-18, -1.000000000000000000, 0.000000000000000000 ) ) ;
#54717=CIRCLE ( 'NONE', #61470, 20.00000000000000000 ) ;
#54753=CARTESIAN_POINT ( 'NONE',  ( 283.3057637310466248, -21.67663200833031922, -3.765392563550209459 ) ) ;
#54819=ORIENTED_EDGE ( 'NONE', *, *, #64391, .F. ) ;
#54862=EDGE_LOOP ( 'NONE', ( #6638, #29764, #39484, #22906 ) ) ;
#54877=VERTEX_POINT ( 'NONE', #64461 ) ;
#54896=CARTESIAN_POINT ( 'NONE',  ( 113.0554507864566318, 21.63937313260594664, 3.971423903130212985 ) ) ;
#54900=LINE ( 'NONE', #19974, #6165 ) ;
#54907=CARTESIAN_POINT ( 'NONE',  ( 100.0000000000000284, 5.000000000000000000, 21.42428528562851753 ) ) ;
#54971=LINE ( 'NONE', #59543, #16938 ) ;
#55102=CARTESIAN_POINT ( 'NONE',  ( 280.0000000000000000, -21.42428528562853529, -4.999999999999990230 ) ) ;
#55630=FACE_OUTER_BOUND ( 'NONE', #54862, .T. ) ;
#55751=DIRECTION ( 'NONE',  ( -1.000000000000000000, -0.000000000000000000, -0.000000000000000000 ) ) ;
#55904=EDGE_CURVE ( 'NONE', #11779, #45015, #20758, .T. ) ;
#55905=VECTOR ( 'NONE', #36695, 1000.000000000000000 ) ;
#56073=CARTESIAN_POINT ( 'NONE',  ( 275.5096892522198573, -21.88944388124440010, 2.223599993928938812 ) ) ;
#56083=CARTESIAN_POINT ( 'NONE',  ( 277.7821011353898939, 21.53668059256674638, -4.493084242282730401 ) ) ;
#56117=DIRECTION ( 'NONE',  ( -1.000000000000000000, -0.000000000000000000, -0.000000000000000000 ) ) ;
#56154=CARTESIAN_POINT ( 'NONE',  ( 284.4935831913008997, -21.89011901571377194, 2.216886222927867856 ) ) ;
#56166=EDGE_LOOP ( 'NONE', ( #27281, #9239 ) ) ;
#56337=CARTESIAN_POINT ( 'NONE',  ( 100.0000000000000284, -5.000000000000000000, 18.50000000000000000 ) ) ;
#56408=CARTESIAN_POINT ( 'NONE',  ( 283.7642062731435431, 21.75126402171896345, -3.307110067226755490 ) ) ;
#56411=CARTESIAN_POINT ( 'NONE',  ( 276.0271074675582099, -21.78879721737672881, -3.053546265906994517 ) ) ;
#56420=CARTESIAN_POINT ( 'NONE',  ( 279.3411025683419666, 21.43200632497276104, -4.967238636669200069 ) ) ;
#56455=AXIS2_PLACEMENT_3D ( 'NONE', #53746, #22445, #11887 ) ;
#56460=CIRCLE ( 'NONE', #50894, 21.99999999999997158 ) ;
#56709=ADVANCED_FACE ( 'NONE', ( #53568 ), #47598, .T. ) ;
#56758=FACE_OUTER_BOUND ( 'NONE', #38768, .T. ) ;
#56762=CARTESIAN_POINT ( 'NONE',  ( 283.9746407525165637, 21.78913134333902590, -3.050900938606339263 ) ) ;
#56814=ORIENTED_EDGE ( 'NONE', *, *, #29727, .F. ) ;
#56845=CARTESIAN_POINT ( 'NONE',  ( 105.6615829231343042, -21.85840048673441771, -2.507220999339062839 ) ) ;
#57014=( GEOMETRIC_REPRESENTATION_CONTEXT ( 3 ) GLOBAL_UNCERTAINTY_ASSIGNED_CONTEXT ( ( #35994 ) ) GLOBAL_UNIT_ASSIGNED_CONTEXT ( ( #33878, #1878, #18382 ) ) REPRESENTATION_CONTEXT ( 'NONE', 'WORKASPACE' ) );
#57026=CARTESIAN_POINT ( 'NONE',  ( 55.00000000000000000, 19.01593100277521131, 6.196318915105386793 ) ) ;
#57039=EDGE_CURVE ( 'NONE', #8739, #37319, #8793, .T. ) ;
#57106=DIRECTION ( 'NONE',  ( -0.000000000000000000, 0.000000000000000000, -1.000000000000000000 ) ) ;
#57112=CARTESIAN_POINT ( 'NONE',  ( 284.7429971699386329, 21.94267019860760470, -1.616224894600692297 ) ) ;
#57116=CARTESIAN_POINT ( 'NONE',  ( 274.9997958498912567, -22.00004639774357074, -0.3283548106454412530 ) ) ;
#57124=DIRECTION ( 'NONE',  ( -0.000000000000000000, 1.000000000000000000, -0.000000000000000000 ) ) ;
#57171=ORIENTED_EDGE ( 'NONE', *, *, #37145, .T. ) ;
#57220=ORIENTED_EDGE ( 'NONE', *, *, #10333, .F. ) ;
#57247=ORIENTED_EDGE ( 'NONE', *, *, #51003, .T. ) ;
#57360=ORIENTED_EDGE ( 'NONE', *, *, #33608, .F. ) ;
#57449=CARTESIAN_POINT ( 'NONE',  ( 280.0000000000000000, 21.42428528562853884, -4.999999999999990230 ) ) ;
#57457=CARTESIAN_POINT ( 'NONE',  ( 105.2647131865113295, 21.94130279673638384, 1.613668875657356283 ) ) ;
#57468=CARTESIAN_POINT ( 'NONE',  ( 290.0000000000000568, 5.000000000000000888, 21.42428528562853529 ) ) ;
#57801=CARTESIAN_POINT ( 'NONE',  ( 106.9495076362458548, 21.63869423720477769, 3.975053342410763246 ) ) ;
#57828=ORIENTED_EDGE ( 'NONE', *, *, #37730, .F. ) ;
#57852=CARTESIAN_POINT ( 'NONE',  ( 290.0000000000000568, 5.000000000000000888, 18.50000000000000000 ) ) ;
#57875=CARTESIAN_POINT ( 'NONE',  ( 106.6971892993744149, -21.67618688890531331, 3.767895544566254085 ) ) ;
#57937=DIRECTION ( 'NONE',  ( 1.000000000000000000, 0.000000000000000000, 0.000000000000000000 ) ) ;
#58071=CARTESIAN_POINT ( 'NONE',  ( 111.6144526446208403, -21.48289790755741890, -4.743601953786281911 ) ) ;
#58080=FACE_OUTER_BOUND ( 'NONE', #53933, .T. ) ;
#58141=CARTESIAN_POINT ( 'NONE',  ( 280.3314448577247049, 21.42428528562853529, 4.999999999999991118 ) ) ;
#58158=STYLED_ITEM ( 'NONE', ( #2217 ), #63029 ) ;
#58175=CARTESIAN_POINT ( 'NONE',  ( 0.000000000000000000, 0.000000000000000000, 0.000000000000000000 ) ) ;
#58475=CARTESIAN_POINT ( 'NONE',  ( 105.2557116016002681, 21.94295192046379128, -1.612329923324939740 ) ) ;
#58717=DIRECTION ( 'NONE',  ( 0.000000000000000000, 0.000000000000000000, 1.000000000000000000 ) ) ;
#58791=ORIENTED_EDGE ( 'NONE', *, *, #60282, .T. ) ;
#58816=CARTESIAN_POINT ( 'NONE',  ( 280.0000000000000000, 21.42428528562853529, 4.999999999999990230 ) ) ;
#58883=LINE ( 'NONE', #21951, #49777 ) ;
#58980=CARTESIAN_POINT ( 'NONE',  ( 400.0000000000000000, 0.000000000000000000, 0.000000000000000000 ) ) ;
#59126=CARTESIAN_POINT ( 'NONE',  ( 110.3314448577247049, 21.42428528562853174, 5.000000000000002665 ) ) ;
#59199=DIRECTION ( 'NONE',  ( -0.000000000000000000, 1.000000000000000000, -0.000000000000000000 ) ) ;
#59206=ORIENTED_EDGE ( 'NONE', *, *, #20573, .F. ) ;
#59311=CARTESIAN_POINT ( 'NONE',  ( 280.0000000000000000, -22.00000000000000000, 4.999999999999990230 ) ) ;
#59476=CARTESIAN_POINT ( 'NONE',  ( 114.9998692468128780, 21.99997028336874294, -0.3318949079940916591 ) ) ;
#59509=CARTESIAN_POINT ( 'NONE',  ( 105.1608908971991809, 21.96390383200032304, -1.300086469598745520 ) ) ;
#59540=CYLINDRICAL_SURFACE ( 'NONE', #4473, 4.999999999999990230 ) ;
#59543=CARTESIAN_POINT ( 'NONE',  ( -1.224646799147352468E-15, 16.00000000000000000, -5.803681084894614095 ) ) ;
#59571=ORIENTED_EDGE ( 'NONE', *, *, #1162, .T. ) ;
#59603=EDGE_CURVE ( 'NONE', #31823, #45015, #50695, .T. ) ;
#59670=ORIENTED_EDGE ( 'NONE', *, *, #63706, .F. ) ;
#59695=VERTEX_POINT ( 'NONE', #7451 ) ;
#59798=VECTOR ( 'NONE', #15362, 1000.000000000000000 ) ;
#59821=CARTESIAN_POINT ( 'NONE',  ( 110.6524747721059754, 21.43176909745610814, -4.968265989321539067 ) ) ;
#59867=CIRCLE ( 'NONE', #23941, 20.00000000000000000 ) ;
#60020=EDGE_CURVE ( 'NONE', #16987, #39848, #40017, .T. ) ;
#60179=CARTESIAN_POINT ( 'NONE',  ( 114.4933711091048281, 21.89007574053286120, 2.217281872662919540 ) ) ;
#60239=DIRECTION ( 'NONE',  ( 0.000000000000000000, 0.000000000000000000, -1.000000000000000000 ) ) ;
#60282=EDGE_CURVE ( 'NONE', #47125, #13157, #26564, .T. ) ;
#60302=DIRECTION ( 'NONE',  ( 0.000000000000000000, 0.000000000000000000, 1.000000000000000000 ) ) ;
#60501=VERTEX_POINT ( 'NONE', #28653 ) ;
#60536=CARTESIAN_POINT ( 'NONE',  ( 113.3080539574503263, 21.67699184046404781, 3.763267418054582869 ) ) ;
#60540=DIRECTION ( 'NONE',  ( 1.000000000000000000, -4.565061778886334783E-18, 0.000000000000000000 ) ) ;
#60659=CARTESIAN_POINT ( 'NONE',  ( 280.0000000000000000, 21.42428528562853529, 4.999999999999990230 ) ) ;
#60823=CARTESIAN_POINT ( 'NONE',  ( 290.0000000000000568, -5.000000000000000888, 18.50000000000000000 ) ) ;
#60831=DIRECTION ( 'NONE',  ( -0.000000000000000000, 1.000000000000000000, -0.000000000000000000 ) ) ;
#60959=DIRECTION ( 'NONE',  ( 0.000000000000000000, 0.000000000000000000, 1.000000000000000000 ) ) ;
#60989=AXIS2_PLACEMENT_3D ( 'NONE', #65585, #17377, #38857 ) ;
#61000=CARTESIAN_POINT ( 'NONE',  ( 280.0000000000000000, -21.42428528562853884, 4.999999999999990230 ) ) ;
#61276=LINE ( 'NONE', #33518, #41193 ) ;
#61349=CARTESIAN_POINT ( 'NONE',  ( 277.7840330814955792, -21.53650026154319619, 4.493931093091628526 ) ) ;
#61357=CARTESIAN_POINT ( 'NONE',  ( 276.2339232178673001, 21.75159641080505679, 3.304888597515802218 ) ) ;
#61438=CARTESIAN_POINT ( 'NONE',  ( 283.0494652463580678, -21.63856170200817530, -3.975743201777058200 ) ) ;
#61470=AXIS2_PLACEMENT_3D ( 'NONE', #58980, #47386, #5181 ) ;
#61489=VERTEX_POINT ( 'NONE', #57468 ) ;
#61529=CARTESIAN_POINT ( 'NONE',  ( -1.224646799147352468E-15, 0.000000000000000000, 20.00000000000000000 ) ) ;
#61650=ORIENTED_EDGE ( 'NONE', *, *, #18507, .T. ) ;
#61685=CARTESIAN_POINT ( 'NONE',  ( 282.5088088673473976, 21.56899521162237576, -4.337361123092371429 ) ) ;
#61688=CARTESIAN_POINT ( 'NONE',  ( 275.2579757425518210, -21.94246241598116143, 1.618793836905497940 ) ) ;
#61693=EDGE_CURVE ( 'NONE', #68664, #29607, #61276, .T. ) ;
#61696=ORIENTED_EDGE ( 'NONE', *, *, #36290, .F. ) ;
#61697=CARTESIAN_POINT ( 'NONE',  ( 275.2557116016002965, 21.94295192046379128, -1.612329923324941516 ) ) ;
#61724=FACE_BOUND ( 'NONE', #19271, .T. ) ;
#61922=AXIS2_PLACEMENT_3D ( 'NONE', #43767, #525, #10724 ) ;
#62035=CARTESIAN_POINT ( 'NONE',  ( 106.2339232178672290, 21.75159641080504969, 3.304888597515779125 ) ) ;
#62468=( NAMED_UNIT ( * ) SI_UNIT ( $, .STERADIAN. ) SOLID_ANGLE_UNIT ( ) );
#62518=ORIENTED_EDGE ( 'NONE', *, *, #49397, .F. ) ;
#62587=DIRECTION ( 'NONE',  ( 1.000000000000000000, 0.000000000000000000, 0.000000000000000000 ) ) ;
#62644=DIRECTION ( 'NONE',  ( -0.000000000000000000, -0.000000000000000000, 1.000000000000000000 ) ) ;
#62664=CARTESIAN_POINT ( 'NONE',  ( 112.5114001799272074, -21.56931564127029688, 4.335727404899796689 ) ) ;
#62742=CARTESIAN_POINT ( 'NONE',  ( 105.6617573822854155, 21.85836566642198520, 2.507523880400407190 ) ) ;
#62842=CARTESIAN_POINT ( 'NONE',  ( -1.224646799147352468E-15, 16.00000000000000000, -5.803681084894614095 ) ) ;
#62870=CARTESIAN_POINT ( 'NONE',  ( 290.0000000000000568, 2.449293598294704935E-15, -19.99999999999997868 ) ) ;
#62925=CARTESIAN_POINT ( 'NONE',  ( 400.0000000000000000, 0.000000000000000000, 20.00000000000000000 ) ) ;
#63001=CARTESIAN_POINT ( 'NONE',  ( 114.8387163486435298, -21.96381563589838493, -1.302408292197374307 ) ) ;
#63029=MANIFOLD_SOLID_BREP ( 'Cut-Extrude4', #24962 ) ;
#63080=SHAPE_REPRESENTATION ( 'shaft', ( #66832 ), #32049 ) ;
#63138=AXIS2_PLACEMENT_3D ( 'NONE', #13361, #34818, #24265 ) ;
#63154=CARTESIAN_POINT ( 'NONE',  ( 106.2372751229154773, -21.75101418369301598, 3.308700176549400851 ) ) ;
#63349=CARTESIAN_POINT ( 'NONE',  ( 112.2220340837702395, -21.53708152545855370, -4.491189304432825047 ) ) ;
#63364=ORIENTED_EDGE ( 'NONE', *, *, #30579, .T. ) ;
#63375=CARTESIAN_POINT ( 'NONE',  ( 400.0000000000000000, 0.000000000000000000, 0.000000000000000000 ) ) ;
#63487=VECTOR ( 'NONE', #24519, 1000.000000000000000 ) ;
#63525=CIRCLE ( 'NONE', #37703, 20.00000000000000000 ) ;
#63674=DIRECTION ( 'NONE',  ( -1.000000000000000000, -0.000000000000000000, -0.000000000000000000 ) ) ;
#63706=EDGE_CURVE ( 'NONE', #45015, #25409, #26770, .T. ) ;
#63712=ORIENTED_EDGE ( 'NONE', *, *, #30224, .T. ) ;
#63784=LINE ( 'NONE', #31763, #3581 ) ;
#63804=DIRECTION ( 'NONE',  ( 0.000000000000000000, 0.000000000000000000, 1.000000000000000000 ) ) ;
#63874=ORIENTED_EDGE ( 'NONE', *, *, #2460, .T. ) ;
#64111=CARTESIAN_POINT ( 'NONE',  ( 105.0320943261246356, 21.99263847259266669, 0.6545153999150219448 ) ) ;
#64288=ORIENTED_EDGE ( 'NONE', *, *, #30579, .F. ) ;
#64391=EDGE_CURVE ( 'NONE', #68664, #45870, #2795, .T. ) ;
#64455=CARTESIAN_POINT ( 'NONE',  ( 104.9998698049113273, 22.00002958979063550, -0.3253397936368049304 ) ) ;
#64461=CARTESIAN_POINT ( 'NONE',  ( 55.00000000000000000, 19.13941707223176181, -5.803681084894614095 ) ) ;
#64465=ORIENTED_EDGE ( 'NONE', *, *, #38007, .T. ) ;
#64496=EDGE_LOOP ( 'NONE', ( #8471, #65141, #66009, #13 ) ) ;
#64547=PRODUCT_CONTEXT ( 'NONE', #43056, 'mechanical' ) ;
#64581=PLANE ( 'NONE',  #12879 ) ;
#64599=LINE ( 'NONE', #59311, #64942 ) ;
#64750=DIRECTION ( 'NONE',  ( -0.000000000000000000, -0.000000000000000000, 1.000000000000000000 ) ) ;
#64768=CARTESIAN_POINT ( 'NONE',  ( 113.0520942216416387, 21.63891660051134380, -3.973857610334890378 ) ) ;
#64789=ORIENTED_EDGE ( 'NONE', *, *, #28685, .F. ) ;
#64801=LINE ( 'NONE', #27500, #55905 ) ;
#64808=CARTESIAN_POINT ( 'NONE',  ( 105.6635354938838844, 21.85802876872917366, -2.510136981039507997 ) ) ;
#64889=DIRECTION ( 'NONE',  ( -1.000000000000000000, -0.000000000000000000, -0.000000000000000000 ) ) ;
#64942=VECTOR ( 'NONE', #32588, 1000.000000000000000 ) ;
#64974=VERTEX_POINT ( 'NONE', #1946 ) ;
#65120=CARTESIAN_POINT ( 'NONE',  ( 110.0000000000000284, 21.42428528562853529, -5.000000000000004441 ) ) ;
#65131=PLANE ( 'NONE',  #16323 ) ;
#65141=ORIENTED_EDGE ( 'NONE', *, *, #43815, .T. ) ;
#65169=PLANE ( 'NONE',  #67570 ) ;
#65318=LINE ( 'NONE', #54036, #41648 ) ;
#65325=CARTESIAN_POINT ( 'NONE',  ( 281.3018128478065023, -21.46140473645479929, 4.838640910132730788 ) ) ;
#65472=CARTESIAN_POINT ( 'NONE',  ( 110.3268469170084245, 21.42428528562853174, -5.000000000000004441 ) ) ;
#65585=CARTESIAN_POINT ( 'NONE',  ( 290.0000000000000568, 5.000000000000000888, 18.50000000000000000 ) ) ;
#65681=CARTESIAN_POINT ( 'NONE',  ( 281.2988829979104821, -21.46124357533057747, -4.839350883597167474 ) ) ;
#65683=ADVANCED_FACE ( 'NONE', ( #58080 ), #32985, .F. ) ;
#65752=DIRECTION ( 'NONE',  ( -1.000000000000000000, 0.000000000000000000, -0.000000000000000000 ) ) ;
#66007=ORIENTED_EDGE ( 'NONE', *, *, #53660, .F. ) ;
#66009=ORIENTED_EDGE ( 'NONE', *, *, #24705, .T. ) ;
#66041=CARTESIAN_POINT ( 'NONE',  ( 281.6144526446208829, -21.48289790755742956, -4.743601953786250824 ) ) ;
#66119=AXIS2_PLACEMENT_3D ( 'NONE', #18746, #28611, #23344 ) ;
#66314=CARTESIAN_POINT ( 'NONE',  ( 276.2331853604025014, 21.75170065437620437, -3.304351318131944826 ) ) ;
#66395=ORIENTED_EDGE ( 'NONE', *, *, #37299, .F. ) ;
#66420=ORIENTED_EDGE ( 'NONE', *, *, #21836, .F. ) ;
#66832=AXIS2_PLACEMENT_3D ( 'NONE', #50530, #44558, #8319 ) ;
#66924=ORIENTED_EDGE ( 'NONE', *, *, #37730, .T. ) ;
#66995=CARTESIAN_POINT ( 'NONE',  ( 278.8631335077134281, -21.45382118812038286, 4.871821213770100023 ) ) ;
#67003=CARTESIAN_POINT ( 'NONE',  ( 275.0326735325356253, 21.99250842598268463, -0.6579281897535153023 ) ) ;
#67034=DIRECTION ( 'NONE',  ( 0.000000000000000000, 0.000000000000000000, 1.000000000000000000 ) ) ;
#67086=CARTESIAN_POINT ( 'NONE',  ( 280.3299582524531388, -21.42428528562853174, -4.999999999999992006 ) ) ;
#67563=DIRECTION ( 'NONE',  ( 1.000000000000000000, 0.000000000000000000, -0.000000000000000000 ) ) ;
#67570=AXIS2_PLACEMENT_3D ( 'NONE', #12401, #54599, #6425 ) ;
#67748=CARTESIAN_POINT ( 'NONE',  ( 105.0330373230561918, -21.99242646597928896, 0.6602422734858272024 ) ) ;
#67918=VECTOR ( 'NONE', #22405, 1000.000000000000000 ) ;
#67947=CARTESIAN_POINT ( 'NONE',  ( 112.2205320413088145, -21.53693364843037372, 4.491889980468759980 ) ) ;
#68098=CARTESIAN_POINT ( 'NONE',  ( 108.3885044869535079, -21.48423713950020897, 4.736025848076682365 ) ) ;
#68221=AXIS2_PLACEMENT_3D ( 'NONE', #45472, #39174, #60959 ) ;
#68288=CARTESIAN_POINT ( 'NONE',  ( 114.7439874972685345, -21.94289037477085813, 1.612903297879166642 ) ) ;
#68359=CARTESIAN_POINT ( 'NONE',  ( 280.3268469170084245, 21.42428528562853529, -4.999999999999990230 ) ) ;
#68366=CARTESIAN_POINT ( 'NONE',  ( 109.3426986656772470, 21.43197803755063902, 4.967354168418953719 ) ) ;
#68430=CARTESIAN_POINT ( 'NONE',  ( 110.0000000000000284, -21.42428528562853529, 5.000000000000004441 ) ) ;
#68491=CIRCLE ( 'NONE', #40423, 19.99999999999997868 ) ;
#68620=CARTESIAN_POINT ( 'NONE',  ( 114.7429429236411238, -21.94266591301279234, -1.615775360921249959 ) ) ;
#68664=VERTEX_POINT ( 'NONE', #33824 ) ;
#68737=EDGE_CURVE ( 'NONE', #54877, #17632, #36429, .T. ) ;
#68759=CARTESIAN_POINT ( 'NONE',  ( 105.0002060648038480, -21.99995316709852489, 0.3345430166890353552 ) ) ;
#68810=LINE ( 'NONE', #48628, #59798 ) ;
#68952=CARTESIAN_POINT ( 'NONE',  ( 110.6590877922806015, -21.43203852822544064, -4.967093445758837156 ) ) ;
#69039=AXIS2_PLACEMENT_3D ( 'NONE', #21700, #241, #22402 ) ;
#69101=CARTESIAN_POINT ( 'NONE',  ( 108.8631335077135418, -21.45382118812038641, 4.871821213770127557 ) ) ;
#69113=CARTESIAN_POINT ( 'NONE',  ( 0.000000000000000000, 2.449293598294705330E-15, -19.99999999999998934 ) ) ;
#69249=ADVANCED_BREP_SHAPE_REPRESENTATION ( '', ( #63029, #66832 ), #32049 ) ;
#69389=ADVANCED_FACE ( 'NONE', ( #54037 ), #27670, .F. ) ;
#69566=DIRECTION ( 'NONE',  ( 0.000000000000000000, 0.000000000000000000, 1.000000000000000000 ) ) ;
ENDSEC;
END-ISO-10303-21;
